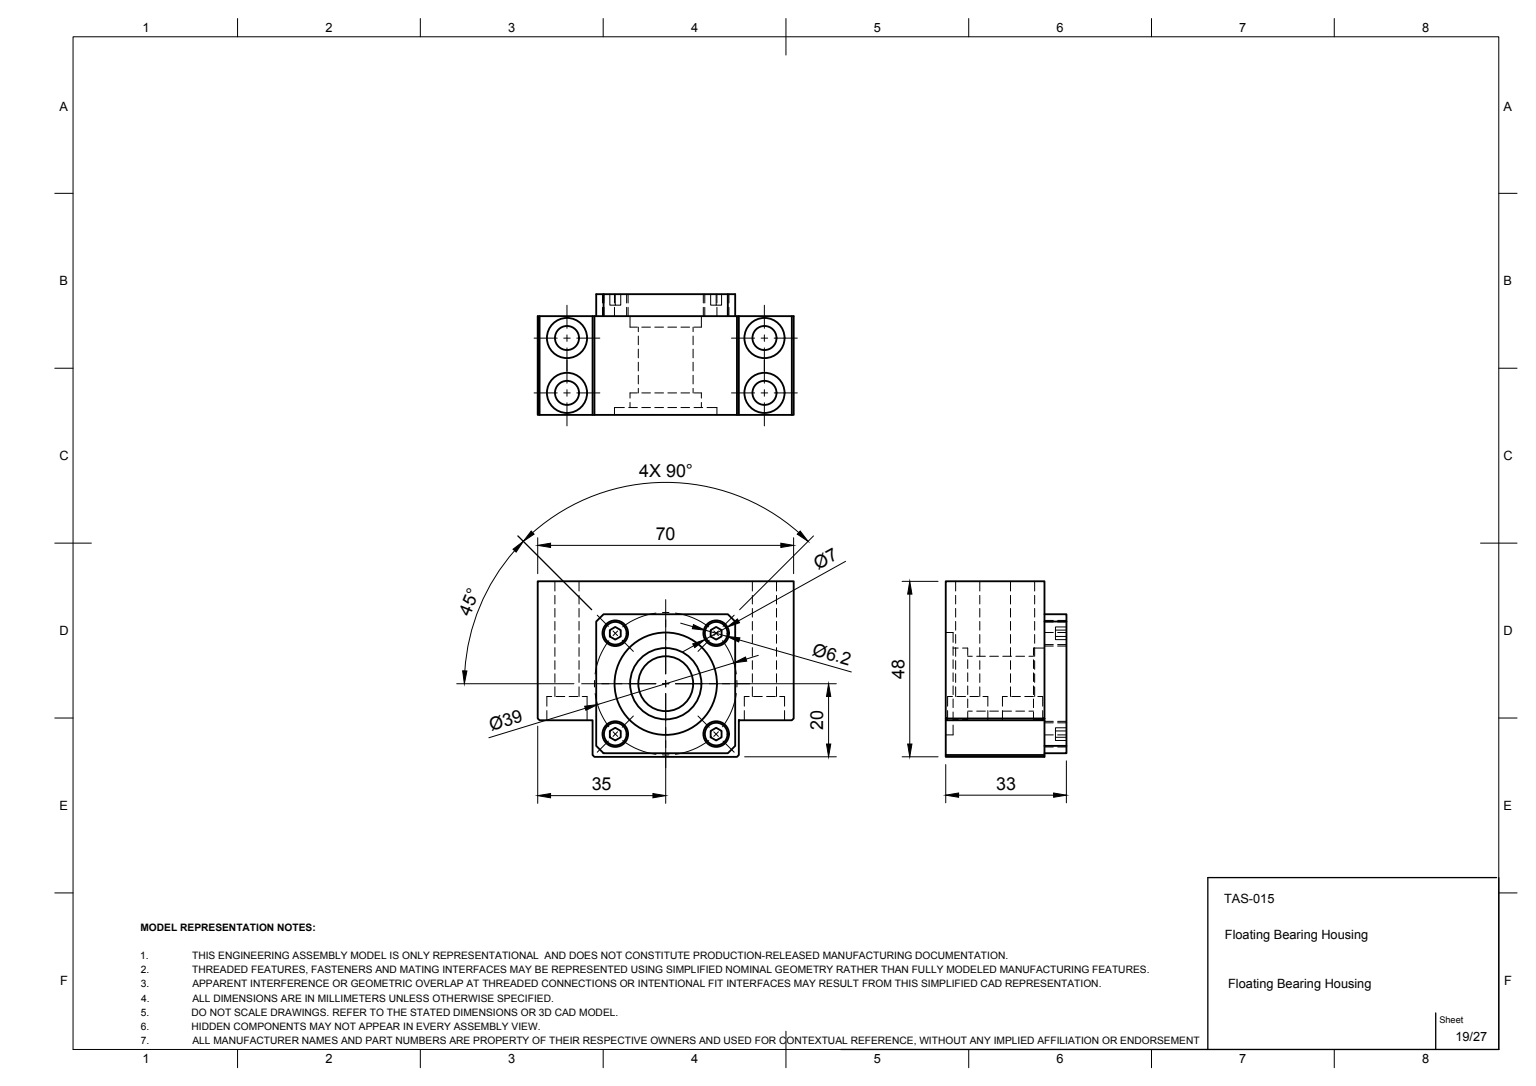
ISO-10303-21;
HEADER;
/* Generated by software containing ST-Developer
 * from STEP Tools, Inc. (www.steptools.com) 
 */

FILE_DESCRIPTION(
/* description */ ('STEP AP214'),
/* implementation_level */ '2;1');

FILE_NAME(
/* name */ 'Floating Bearing Housing.step',
/* time_stamp */ '2026-11-15T14:49:54-08:00',
/* author */ (''),
/* organization */ (''),
/* preprocessor_version */ 'ST-DEVELOPER v20.2',
/* originating_system */ 'Autodesk Translation Framework v15.17.0.0',
/* authorisation */ '');

FILE_SCHEMA (('AUTOMOTIVE_DESIGN { 1 0 10303 214 3 1 1 }'));
ENDSEC;

DATA;
#10=MECHANICAL_DESIGN_GEOMETRIC_PRESENTATION_REPRESENTATION('',(#1111),#66721);
#1049=SHAPE_REPRESENTATION_RELATIONSHIP('SRR','None',#66910,#1080);
#1080=ADVANCED_BREP_SHAPE_REPRESENTATION('',(#1146),#66701);
#1111=STYLED_ITEM('',(#67095),#1146);
#1146=MANIFOLD_SOLID_BREP('Body1',#25677);
#1342=FACE_BOUND('',#4614,.T.);
#1343=FACE_BOUND('',#4616,.T.);
#1344=FACE_BOUND('',#4618,.T.);
#1345=FACE_BOUND('',#4620,.T.);
#1346=FACE_BOUND('',#4622,.T.);
#1347=FACE_BOUND('',#4624,.T.);
#1348=FACE_BOUND('',#4625,.T.);
#1349=FACE_BOUND('',#4629,.T.);
#1350=FACE_BOUND('',#4630,.T.);
#1351=FACE_BOUND('',#4631,.T.);
#1352=FACE_BOUND('',#4632,.T.);
#1353=FACE_BOUND('',#4636,.T.);
#1354=FACE_BOUND('',#4637,.T.);
#1355=FACE_BOUND('',#4644,.T.);
#1356=FACE_BOUND('',#4646,.T.);
#1357=FACE_BOUND('',#4648,.T.);
#1358=FACE_BOUND('',#4650,.T.);
#1359=FACE_BOUND('',#4652,.T.);
#1360=FACE_BOUND('',#4654,.T.);
#1361=FACE_BOUND('',#4655,.T.);
#1362=FACE_BOUND('',#4656,.T.);
#1363=FACE_BOUND('',#4657,.T.);
#1364=FACE_BOUND('',#4658,.T.);
#1365=FACE_BOUND('',#4668,.T.);
#1366=FACE_BOUND('',#4670,.T.);
#1367=FACE_BOUND('',#4672,.T.);
#1368=FACE_BOUND('',#4674,.T.);
#1369=FACE_BOUND('',#4704,.T.);
#1370=FACE_BOUND('',#4706,.T.);
#1371=FACE_BOUND('',#4708,.T.);
#1372=FACE_BOUND('',#4710,.T.);
#1915=PLANE('',#27535);
#1916=PLANE('',#27536);
#1917=PLANE('',#27537);
#1918=PLANE('',#27538);
#1919=PLANE('',#27539);
#1920=PLANE('',#27540);
#1921=PLANE('',#27541);
#1922=PLANE('',#27542);
#1923=PLANE('',#27543);
#1924=PLANE('',#27544);
#1925=PLANE('',#27545);
#1926=PLANE('',#27546);
#1927=PLANE('',#27547);
#1928=PLANE('',#27548);
#1929=PLANE('',#27549);
#1930=PLANE('',#27550);
#1931=PLANE('',#27551);
#1932=PLANE('',#27552);
#1933=PLANE('',#27553);
#1934=PLANE('',#27554);
#1935=PLANE('',#27555);
#1936=PLANE('',#27556);
#1937=PLANE('',#27557);
#1938=PLANE('',#27558);
#1939=PLANE('',#27559);
#1940=PLANE('',#27560);
#1941=PLANE('',#27561);
#1942=PLANE('',#27562);
#1943=PLANE('',#27563);
#1944=PLANE('',#27564);
#1945=PLANE('',#27565);
#1946=PLANE('',#27566);
#1947=PLANE('',#27567);
#1948=PLANE('',#27568);
#1949=PLANE('',#27569);
#1950=PLANE('',#27570);
#1951=PLANE('',#27571);
#1952=PLANE('',#27572);
#1953=PLANE('',#27573);
#1954=PLANE('',#27574);
#1955=PLANE('',#27575);
#1956=PLANE('',#27576);
#1957=PLANE('',#27577);
#1958=PLANE('',#27578);
#1959=PLANE('',#27579);
#1960=PLANE('',#27580);
#1961=PLANE('',#27581);
#1962=PLANE('',#27582);
#1963=PLANE('',#27583);
#1964=PLANE('',#27584);
#1965=PLANE('',#27585);
#1966=PLANE('',#27586);
#1967=PLANE('',#27587);
#1968=PLANE('',#27588);
#1969=PLANE('',#27589);
#1970=PLANE('',#27590);
#1971=PLANE('',#27591);
#1972=PLANE('',#27592);
#1973=PLANE('',#27593);
#1974=PLANE('',#27594);
#1975=PLANE('',#27595);
#1976=PLANE('',#27596);
#1977=PLANE('',#27597);
#1978=PLANE('',#27598);
#1979=PLANE('',#27599);
#1980=PLANE('',#27600);
#1981=PLANE('',#27601);
#2976=FACE_OUTER_BOUND('',#4592,.T.);
#2977=FACE_OUTER_BOUND('',#4593,.T.);
#2978=FACE_OUTER_BOUND('',#4594,.T.);
#2979=FACE_OUTER_BOUND('',#4595,.T.);
#2980=FACE_OUTER_BOUND('',#4596,.T.);
#2981=FACE_OUTER_BOUND('',#4597,.T.);
#2982=FACE_OUTER_BOUND('',#4598,.T.);
#2983=FACE_OUTER_BOUND('',#4599,.T.);
#2984=FACE_OUTER_BOUND('',#4600,.T.);
#2985=FACE_OUTER_BOUND('',#4601,.T.);
#2986=FACE_OUTER_BOUND('',#4602,.T.);
#2987=FACE_OUTER_BOUND('',#4603,.T.);
#2988=FACE_OUTER_BOUND('',#4604,.T.);
#2989=FACE_OUTER_BOUND('',#4605,.T.);
#2990=FACE_OUTER_BOUND('',#4606,.T.);
#2991=FACE_OUTER_BOUND('',#4607,.T.);
#2992=FACE_OUTER_BOUND('',#4608,.T.);
#2993=FACE_OUTER_BOUND('',#4609,.T.);
#2994=FACE_OUTER_BOUND('',#4610,.T.);
#2995=FACE_OUTER_BOUND('',#4611,.T.);
#2996=FACE_OUTER_BOUND('',#4612,.T.);
#2997=FACE_OUTER_BOUND('',#4613,.T.);
#2998=FACE_OUTER_BOUND('',#4615,.T.);
#2999=FACE_OUTER_BOUND('',#4617,.T.);
#3000=FACE_OUTER_BOUND('',#4619,.T.);
#3001=FACE_OUTER_BOUND('',#4621,.T.);
#3002=FACE_OUTER_BOUND('',#4623,.T.);
#3003=FACE_OUTER_BOUND('',#4626,.T.);
#3004=FACE_OUTER_BOUND('',#4627,.T.);
#3005=FACE_OUTER_BOUND('',#4628,.T.);
#3006=FACE_OUTER_BOUND('',#4633,.T.);
#3007=FACE_OUTER_BOUND('',#4634,.T.);
#3008=FACE_OUTER_BOUND('',#4635,.T.);
#3009=FACE_OUTER_BOUND('',#4638,.T.);
#3010=FACE_OUTER_BOUND('',#4639,.T.);
#3011=FACE_OUTER_BOUND('',#4640,.T.);
#3012=FACE_OUTER_BOUND('',#4641,.T.);
#3013=FACE_OUTER_BOUND('',#4642,.T.);
#3014=FACE_OUTER_BOUND('',#4643,.T.);
#3015=FACE_OUTER_BOUND('',#4645,.T.);
#3016=FACE_OUTER_BOUND('',#4647,.T.);
#3017=FACE_OUTER_BOUND('',#4649,.T.);
#3018=FACE_OUTER_BOUND('',#4651,.T.);
#3019=FACE_OUTER_BOUND('',#4653,.T.);
#3020=FACE_OUTER_BOUND('',#4659,.T.);
#3021=FACE_OUTER_BOUND('',#4660,.T.);
#3022=FACE_OUTER_BOUND('',#4661,.T.);
#3023=FACE_OUTER_BOUND('',#4662,.T.);
#3024=FACE_OUTER_BOUND('',#4663,.T.);
#3025=FACE_OUTER_BOUND('',#4664,.T.);
#3026=FACE_OUTER_BOUND('',#4665,.T.);
#3027=FACE_OUTER_BOUND('',#4666,.T.);
#3028=FACE_OUTER_BOUND('',#4667,.T.);
#3029=FACE_OUTER_BOUND('',#4669,.T.);
#3030=FACE_OUTER_BOUND('',#4671,.T.);
#3031=FACE_OUTER_BOUND('',#4673,.T.);
#3032=FACE_OUTER_BOUND('',#4675,.T.);
#3033=FACE_OUTER_BOUND('',#4676,.T.);
#3034=FACE_OUTER_BOUND('',#4677,.T.);
#3035=FACE_OUTER_BOUND('',#4678,.T.);
#3036=FACE_OUTER_BOUND('',#4679,.T.);
#3037=FACE_OUTER_BOUND('',#4680,.T.);
#3038=FACE_OUTER_BOUND('',#4681,.T.);
#3039=FACE_OUTER_BOUND('',#4682,.T.);
#3040=FACE_OUTER_BOUND('',#4683,.T.);
#3041=FACE_OUTER_BOUND('',#4684,.T.);
#3042=FACE_OUTER_BOUND('',#4685,.T.);
#3043=FACE_OUTER_BOUND('',#4686,.T.);
#3044=FACE_OUTER_BOUND('',#4687,.T.);
#3045=FACE_OUTER_BOUND('',#4688,.T.);
#3046=FACE_OUTER_BOUND('',#4689,.T.);
#3047=FACE_OUTER_BOUND('',#4690,.T.);
#3048=FACE_OUTER_BOUND('',#4691,.T.);
#3049=FACE_OUTER_BOUND('',#4692,.T.);
#3050=FACE_OUTER_BOUND('',#4693,.T.);
#3051=FACE_OUTER_BOUND('',#4694,.T.);
#3052=FACE_OUTER_BOUND('',#4695,.T.);
#3053=FACE_OUTER_BOUND('',#4696,.T.);
#3054=FACE_OUTER_BOUND('',#4697,.T.);
#3055=FACE_OUTER_BOUND('',#4698,.T.);
#3056=FACE_OUTER_BOUND('',#4699,.T.);
#3057=FACE_OUTER_BOUND('',#4700,.T.);
#3058=FACE_OUTER_BOUND('',#4701,.T.);
#3059=FACE_OUTER_BOUND('',#4702,.T.);
#3060=FACE_OUTER_BOUND('',#4703,.T.);
#3061=FACE_OUTER_BOUND('',#4705,.T.);
#3062=FACE_OUTER_BOUND('',#4707,.T.);
#3063=FACE_OUTER_BOUND('',#4709,.T.);
#4592=EDGE_LOOP('',(#20414,#20415,#20416,#20417));
#4593=EDGE_LOOP('',(#20418,#20419,#20420,#20421));
#4594=EDGE_LOOP('',(#20422,#20423,#20424,#20425));
#4595=EDGE_LOOP('',(#20426,#20427,#20428,#20429));
#4596=EDGE_LOOP('',(#20430,#20431,#20432,#20433));
#4597=EDGE_LOOP('',(#20434,#20435,#20436,#20437));
#4598=EDGE_LOOP('',(#20438,#20439,#20440,#20441));
#4599=EDGE_LOOP('',(#20442,#20443,#20444,#20445));
#4600=EDGE_LOOP('',(#20446,#20447,#20448,#20449));
#4601=EDGE_LOOP('',(#20450,#20451,#20452,#20453));
#4602=EDGE_LOOP('',(#20454,#20455,#20456,#20457));
#4603=EDGE_LOOP('',(#20458,#20459,#20460,#20461));
#4604=EDGE_LOOP('',(#20462,#20463,#20464,#20465));
#4605=EDGE_LOOP('',(#20466,#20467,#20468,#20469));
#4606=EDGE_LOOP('',(#20470,#20471,#20472,#20473));
#4607=EDGE_LOOP('',(#20474,#20475,#20476,#20477));
#4608=EDGE_LOOP('',(#20478,#20479,#20480,#20481));
#4609=EDGE_LOOP('',(#20482,#20483,#20484,#20485));
#4610=EDGE_LOOP('',(#20486,#20487,#20488,#20489));
#4611=EDGE_LOOP('',(#20490,#20491,#20492,#20493));
#4612=EDGE_LOOP('',(#20494,#20495,#20496,#20497));
#4613=EDGE_LOOP('',(#20498));
#4614=EDGE_LOOP('',(#20499));
#4615=EDGE_LOOP('',(#20500));
#4616=EDGE_LOOP('',(#20501));
#4617=EDGE_LOOP('',(#20502));
#4618=EDGE_LOOP('',(#20503));
#4619=EDGE_LOOP('',(#20504));
#4620=EDGE_LOOP('',(#20505));
#4621=EDGE_LOOP('',(#20506,#20507,#20508,#20509,#20510,#20511,#20512,#20513,
#20514,#20515,#20516,#20517));
#4622=EDGE_LOOP('',(#20518,#20519,#20520,#20521,#20522,#20523,#20524,#20525));
#4623=EDGE_LOOP('',(#20526,#20527,#20528,#20529));
#4624=EDGE_LOOP('',(#20530));
#4625=EDGE_LOOP('',(#20531));
#4626=EDGE_LOOP('',(#20532,#20533,#20534,#20535));
#4627=EDGE_LOOP('',(#20536,#20537,#20538,#20539));
#4628=EDGE_LOOP('',(#20540,#20541,#20542,#20543));
#4629=EDGE_LOOP('',(#20544));
#4630=EDGE_LOOP('',(#20545));
#4631=EDGE_LOOP('',(#20546));
#4632=EDGE_LOOP('',(#20547));
#4633=EDGE_LOOP('',(#20548,#20549,#20550,#20551));
#4634=EDGE_LOOP('',(#20552,#20553,#20554,#20555));
#4635=EDGE_LOOP('',(#20556,#20557,#20558,#20559));
#4636=EDGE_LOOP('',(#20560));
#4637=EDGE_LOOP('',(#20561));
#4638=EDGE_LOOP('',(#20562,#20563,#20564,#20565));
#4639=EDGE_LOOP('',(#20566,#20567,#20568,#20569));
#4640=EDGE_LOOP('',(#20570,#20571,#20572,#20573));
#4641=EDGE_LOOP('',(#20574,#20575,#20576,#20577));
#4642=EDGE_LOOP('',(#20578,#20579,#20580,#20581));
#4643=EDGE_LOOP('',(#20582,#20583,#20584,#20585,#20586,#20587,#20588,#20589,
#20590,#20591,#20592,#20593));
#4644=EDGE_LOOP('',(#20594));
#4645=EDGE_LOOP('',(#20595));
#4646=EDGE_LOOP('',(#20596));
#4647=EDGE_LOOP('',(#20597));
#4648=EDGE_LOOP('',(#20598));
#4649=EDGE_LOOP('',(#20599));
#4650=EDGE_LOOP('',(#20600));
#4651=EDGE_LOOP('',(#20601));
#4652=EDGE_LOOP('',(#20602));
#4653=EDGE_LOOP('',(#20603,#20604,#20605,#20606,#20607,#20608,#20609,#20610));
#4654=EDGE_LOOP('',(#20611));
#4655=EDGE_LOOP('',(#20612));
#4656=EDGE_LOOP('',(#20613));
#4657=EDGE_LOOP('',(#20614));
#4658=EDGE_LOOP('',(#20615));
#4659=EDGE_LOOP('',(#20616,#20617,#20618,#20619));
#4660=EDGE_LOOP('',(#20620,#20621,#20622,#20623));
#4661=EDGE_LOOP('',(#20624,#20625,#20626,#20627));
#4662=EDGE_LOOP('',(#20628,#20629,#20630,#20631));
#4663=EDGE_LOOP('',(#20632,#20633,#20634,#20635));
#4664=EDGE_LOOP('',(#20636,#20637,#20638,#20639));
#4665=EDGE_LOOP('',(#20640,#20641,#20642,#20643));
#4666=EDGE_LOOP('',(#20644,#20645,#20646,#20647));
#4667=EDGE_LOOP('',(#20648));
#4668=EDGE_LOOP('',(#20649,#20650,#20651,#20652,#20653,#20654));
#4669=EDGE_LOOP('',(#20655));
#4670=EDGE_LOOP('',(#20656,#20657,#20658,#20659,#20660,#20661));
#4671=EDGE_LOOP('',(#20662));
#4672=EDGE_LOOP('',(#20663,#20664,#20665,#20666,#20667,#20668));
#4673=EDGE_LOOP('',(#20669));
#4674=EDGE_LOOP('',(#20670,#20671,#20672,#20673,#20674,#20675));
#4675=EDGE_LOOP('',(#20676,#20677,#20678,#20679));
#4676=EDGE_LOOP('',(#20680,#20681,#20682,#20683));
#4677=EDGE_LOOP('',(#20684,#20685,#20686,#20687));
#4678=EDGE_LOOP('',(#20688,#20689,#20690,#20691));
#4679=EDGE_LOOP('',(#20692,#20693,#20694,#20695));
#4680=EDGE_LOOP('',(#20696,#20697,#20698,#20699));
#4681=EDGE_LOOP('',(#20700,#20701,#20702,#20703,#20704,#20705));
#4682=EDGE_LOOP('',(#20706,#20707,#20708,#20709));
#4683=EDGE_LOOP('',(#20710,#20711,#20712,#20713));
#4684=EDGE_LOOP('',(#20714,#20715,#20716,#20717));
#4685=EDGE_LOOP('',(#20718,#20719,#20720,#20721));
#4686=EDGE_LOOP('',(#20722,#20723,#20724,#20725));
#4687=EDGE_LOOP('',(#20726,#20727,#20728,#20729));
#4688=EDGE_LOOP('',(#20730,#20731,#20732,#20733,#20734,#20735));
#4689=EDGE_LOOP('',(#20736,#20737,#20738,#20739));
#4690=EDGE_LOOP('',(#20740,#20741,#20742,#20743));
#4691=EDGE_LOOP('',(#20744,#20745,#20746,#20747));
#4692=EDGE_LOOP('',(#20748,#20749,#20750,#20751));
#4693=EDGE_LOOP('',(#20752,#20753,#20754,#20755));
#4694=EDGE_LOOP('',(#20756,#20757,#20758,#20759));
#4695=EDGE_LOOP('',(#20760,#20761,#20762,#20763,#20764,#20765));
#4696=EDGE_LOOP('',(#20766,#20767,#20768,#20769));
#4697=EDGE_LOOP('',(#20770,#20771,#20772,#20773));
#4698=EDGE_LOOP('',(#20774,#20775,#20776,#20777));
#4699=EDGE_LOOP('',(#20778,#20779,#20780,#20781));
#4700=EDGE_LOOP('',(#20782,#20783,#20784,#20785));
#4701=EDGE_LOOP('',(#20786,#20787,#20788,#20789));
#4702=EDGE_LOOP('',(#20790,#20791,#20792,#20793,#20794,#20795));
#4703=EDGE_LOOP('',(#20796));
#4704=EDGE_LOOP('',(#20797));
#4705=EDGE_LOOP('',(#20798));
#4706=EDGE_LOOP('',(#20799));
#4707=EDGE_LOOP('',(#20800));
#4708=EDGE_LOOP('',(#20801));
#4709=EDGE_LOOP('',(#20802));
#4710=EDGE_LOOP('',(#20803));
#6658=LINE('',#40429,#8647);
#6659=LINE('',#40435,#8648);
#6660=LINE('',#40441,#8649);
#6661=LINE('',#40447,#8650);
#6662=LINE('',#40453,#8651);
#6663=LINE('',#40459,#8652);
#6664=LINE('',#40465,#8653);
#6665=LINE('',#40471,#8654);
#6666=LINE('',#40477,#8655);
#6667=LINE('',#40483,#8656);
#6668=LINE('',#40489,#8657);
#6669=LINE('',#40495,#8658);
#6670=LINE('',#40501,#8659);
#6671=LINE('',#40507,#8660);
#6672=LINE('',#40513,#8661);
#6673=LINE('',#40519,#8662);
#6674=LINE('',#40525,#8663);
#6675=LINE('',#40531,#8664);
#6676=LINE('',#40537,#8665);
#6677=LINE('',#40543,#8666);
#6678=LINE('',#40549,#8667);
#6679=LINE('',#40558,#8668);
#6680=LINE('',#40560,#8669);
#6681=LINE('',#40562,#8670);
#6682=LINE('',#40564,#8671);
#6683=LINE('',#40566,#8672);
#6684=LINE('',#40568,#8673);
#6685=LINE('',#40570,#8674);
#6686=LINE('',#40572,#8675);
#6687=LINE('',#40574,#8676);
#6688=LINE('',#40576,#8677);
#6689=LINE('',#40578,#8678);
#6690=LINE('',#40579,#8679);
#6691=LINE('',#40582,#8680);
#6692=LINE('',#40584,#8681);
#6693=LINE('',#40586,#8682);
#6694=LINE('',#40588,#8683);
#6695=LINE('',#40590,#8684);
#6696=LINE('',#40592,#8685);
#6697=LINE('',#40594,#8686);
#6698=LINE('',#40595,#8687);
#6699=LINE('',#40599,#8688);
#6700=LINE('',#40600,#8689);
#6701=LINE('',#40601,#8690);
#6702=LINE('',#40604,#8691);
#6703=LINE('',#40605,#8692);
#6704=LINE('',#40608,#8693);
#6705=LINE('',#40609,#8694);
#6706=LINE('',#40612,#8695);
#6707=LINE('',#40613,#8696);
#6708=LINE('',#40616,#8697);
#6709=LINE('',#40617,#8698);
#6710=LINE('',#40620,#8699);
#6711=LINE('',#40621,#8700);
#6712=LINE('',#40624,#8701);
#6713=LINE('',#40625,#8702);
#6714=LINE('',#40628,#8703);
#6715=LINE('',#40629,#8704);
#6716=LINE('',#40632,#8705);
#6717=LINE('',#40633,#8706);
#6718=LINE('',#40636,#8707);
#6719=LINE('',#40637,#8708);
#6720=LINE('',#40640,#8709);
#6721=LINE('',#40641,#8710);
#6722=LINE('',#40643,#8711);
#6723=LINE('',#40652,#8712);
#6724=LINE('',#40654,#8713);
#6725=LINE('',#40656,#8714);
#6726=LINE('',#40658,#8715);
#6727=LINE('',#40660,#8716);
#6728=LINE('',#40662,#8717);
#6729=LINE('',#40664,#8718);
#6730=LINE('',#40665,#8719);
#6731=LINE('',#40667,#8720);
#6732=LINE('',#40668,#8721);
#6733=LINE('',#40670,#8722);
#6734=LINE('',#40672,#8723);
#6735=LINE('',#40674,#8724);
#6736=LINE('',#40676,#8725);
#6737=LINE('',#40678,#8726);
#6738=LINE('',#40680,#8727);
#6739=LINE('',#40685,#8728);
#6740=LINE('',#40687,#8729);
#6741=LINE('',#40689,#8730);
#6742=LINE('',#40691,#8731);
#6743=LINE('',#40693,#8732);
#6744=LINE('',#40694,#8733);
#6745=LINE('',#40698,#8734);
#6746=LINE('',#40700,#8735);
#6747=LINE('',#40702,#8736);
#6748=LINE('',#40704,#8737);
#6749=LINE('',#40706,#8738);
#6750=LINE('',#40707,#8739);
#6751=LINE('',#40711,#8740);
#6752=LINE('',#40713,#8741);
#6753=LINE('',#40715,#8742);
#6754=LINE('',#40717,#8743);
#6755=LINE('',#40719,#8744);
#6756=LINE('',#40720,#8745);
#6757=LINE('',#40724,#8746);
#6758=LINE('',#40726,#8747);
#6759=LINE('',#40728,#8748);
#6760=LINE('',#40730,#8749);
#6761=LINE('',#40732,#8750);
#6762=LINE('',#40733,#8751);
#6763=LINE('',#40736,#8752);
#6764=LINE('',#40738,#8753);
#6765=LINE('',#40739,#8754);
#6766=LINE('',#40742,#8755);
#6767=LINE('',#40743,#8756);
#6768=LINE('',#40746,#8757);
#6769=LINE('',#40747,#8758);
#6770=LINE('',#40750,#8759);
#6771=LINE('',#40751,#8760);
#6772=LINE('',#40754,#8761);
#6773=LINE('',#40755,#8762);
#6774=LINE('',#40757,#8763);
#6775=LINE('',#40761,#8764);
#6776=LINE('',#40763,#8765);
#6777=LINE('',#40764,#8766);
#6778=LINE('',#40767,#8767);
#6779=LINE('',#40768,#8768);
#6780=LINE('',#40771,#8769);
#6781=LINE('',#40772,#8770);
#6782=LINE('',#40775,#8771);
#6783=LINE('',#40776,#8772);
#6784=LINE('',#40779,#8773);
#6785=LINE('',#40780,#8774);
#6786=LINE('',#40782,#8775);
#6787=LINE('',#40786,#8776);
#6788=LINE('',#40788,#8777);
#6789=LINE('',#40789,#8778);
#6790=LINE('',#40792,#8779);
#6791=LINE('',#40793,#8780);
#6792=LINE('',#40796,#8781);
#6793=LINE('',#40797,#8782);
#6794=LINE('',#40800,#8783);
#6795=LINE('',#40801,#8784);
#6796=LINE('',#40804,#8785);
#6797=LINE('',#40805,#8786);
#6798=LINE('',#40807,#8787);
#6799=LINE('',#40811,#8788);
#6800=LINE('',#40813,#8789);
#6801=LINE('',#40814,#8790);
#6802=LINE('',#40817,#8791);
#6803=LINE('',#40818,#8792);
#6804=LINE('',#40821,#8793);
#6805=LINE('',#40822,#8794);
#6806=LINE('',#40825,#8795);
#6807=LINE('',#40826,#8796);
#6808=LINE('',#40829,#8797);
#6809=LINE('',#40830,#8798);
#6810=LINE('',#40832,#8799);
#8647=VECTOR('',#32797,14.);
#8648=VECTOR('',#32804,9.75);
#8649=VECTOR('',#32811,7.5);
#8650=VECTOR('',#32818,9.75);
#8651=VECTOR('',#32825,14.);
#8652=VECTOR('',#32832,3.1);
#8653=VECTOR('',#32839,3.1);
#8654=VECTOR('',#32846,3.1);
#8655=VECTOR('',#32853,3.1);
#8656=VECTOR('',#32860,3.50000000000001);
#8657=VECTOR('',#32867,3.5);
#8658=VECTOR('',#32874,3.50000000000001);
#8659=VECTOR('',#32881,3.50000000000001);
#8660=VECTOR('',#32888,5.5);
#8661=VECTOR('',#32895,3.3);
#8662=VECTOR('',#32902,5.5);
#8663=VECTOR('',#32909,3.3);
#8664=VECTOR('',#32916,5.5);
#8665=VECTOR('',#32923,3.3);
#8666=VECTOR('',#32930,5.5);
#8667=VECTOR('',#32937,3.3);
#8668=VECTOR('',#32950,1000.);
#8669=VECTOR('',#32951,1000.);
#8670=VECTOR('',#32952,1000.);
#8671=VECTOR('',#32953,1000.);
#8672=VECTOR('',#32954,1000.);
#8673=VECTOR('',#32955,1000.);
#8674=VECTOR('',#32956,1000.);
#8675=VECTOR('',#32957,1000.);
#8676=VECTOR('',#32958,1000.);
#8677=VECTOR('',#32959,1000.);
#8678=VECTOR('',#32960,1000.);
#8679=VECTOR('',#32961,1000.);
#8680=VECTOR('',#32962,1000.);
#8681=VECTOR('',#32963,1000.);
#8682=VECTOR('',#32964,1000.);
#8683=VECTOR('',#32965,1000.);
#8684=VECTOR('',#32966,1000.);
#8685=VECTOR('',#32967,1000.);
#8686=VECTOR('',#32968,1000.);
#8687=VECTOR('',#32969,1000.);
#8688=VECTOR('',#32972,1000.);
#8689=VECTOR('',#32973,1000.);
#8690=VECTOR('',#32974,1000.);
#8691=VECTOR('',#32977,1000.);
#8692=VECTOR('',#32978,1000.);
#8693=VECTOR('',#32981,1000.);
#8694=VECTOR('',#32982,1000.);
#8695=VECTOR('',#32985,1000.);
#8696=VECTOR('',#32986,1000.);
#8697=VECTOR('',#32989,1000.);
#8698=VECTOR('',#32990,1000.);
#8699=VECTOR('',#32993,1000.);
#8700=VECTOR('',#32994,1000.);
#8701=VECTOR('',#32997,1000.);
#8702=VECTOR('',#32998,1000.);
#8703=VECTOR('',#33001,1000.);
#8704=VECTOR('',#33002,1000.);
#8705=VECTOR('',#33005,1000.);
#8706=VECTOR('',#33006,1000.);
#8707=VECTOR('',#33009,1000.);
#8708=VECTOR('',#33010,1000.);
#8709=VECTOR('',#33013,1000.);
#8710=VECTOR('',#33014,1000.);
#8711=VECTOR('',#33017,1000.);
#8712=VECTOR('',#33030,1000.);
#8713=VECTOR('',#33031,1000.);
#8714=VECTOR('',#33032,1000.);
#8715=VECTOR('',#33033,1000.);
#8716=VECTOR('',#33034,1000.);
#8717=VECTOR('',#33035,1000.);
#8718=VECTOR('',#33036,1000.);
#8719=VECTOR('',#33037,1000.);
#8720=VECTOR('',#33040,1000.);
#8721=VECTOR('',#33041,1000.);
#8722=VECTOR('',#33044,1000.);
#8723=VECTOR('',#33047,1000.);
#8724=VECTOR('',#33050,1000.);
#8725=VECTOR('',#33053,1000.);
#8726=VECTOR('',#33056,1000.);
#8727=VECTOR('',#33059,1000.);
#8728=VECTOR('',#33064,1000.);
#8729=VECTOR('',#33065,1000.);
#8730=VECTOR('',#33066,1000.);
#8731=VECTOR('',#33067,1000.);
#8732=VECTOR('',#33068,1000.);
#8733=VECTOR('',#33069,1000.);
#8734=VECTOR('',#33072,1000.);
#8735=VECTOR('',#33073,1000.);
#8736=VECTOR('',#33074,1000.);
#8737=VECTOR('',#33075,1000.);
#8738=VECTOR('',#33076,1000.);
#8739=VECTOR('',#33077,1000.);
#8740=VECTOR('',#33080,1000.);
#8741=VECTOR('',#33081,1000.);
#8742=VECTOR('',#33082,1000.);
#8743=VECTOR('',#33083,1000.);
#8744=VECTOR('',#33084,1000.);
#8745=VECTOR('',#33085,1000.);
#8746=VECTOR('',#33088,1000.);
#8747=VECTOR('',#33089,1000.);
#8748=VECTOR('',#33090,1000.);
#8749=VECTOR('',#33091,1000.);
#8750=VECTOR('',#33092,1000.);
#8751=VECTOR('',#33093,1000.);
#8752=VECTOR('',#33096,1000.);
#8753=VECTOR('',#33097,1000.);
#8754=VECTOR('',#33098,1000.);
#8755=VECTOR('',#33101,1000.);
#8756=VECTOR('',#33102,1000.);
#8757=VECTOR('',#33105,1000.);
#8758=VECTOR('',#33106,1000.);
#8759=VECTOR('',#33109,1000.);
#8760=VECTOR('',#33110,1000.);
#8761=VECTOR('',#33113,1000.);
#8762=VECTOR('',#33114,1000.);
#8763=VECTOR('',#33117,1000.);
#8764=VECTOR('',#33122,1000.);
#8765=VECTOR('',#33123,1000.);
#8766=VECTOR('',#33124,1000.);
#8767=VECTOR('',#33127,1000.);
#8768=VECTOR('',#33128,1000.);
#8769=VECTOR('',#33131,1000.);
#8770=VECTOR('',#33132,1000.);
#8771=VECTOR('',#33135,1000.);
#8772=VECTOR('',#33136,1000.);
#8773=VECTOR('',#33139,1000.);
#8774=VECTOR('',#33140,1000.);
#8775=VECTOR('',#33143,1000.);
#8776=VECTOR('',#33148,1000.);
#8777=VECTOR('',#33149,1000.);
#8778=VECTOR('',#33150,1000.);
#8779=VECTOR('',#33153,1000.);
#8780=VECTOR('',#33154,1000.);
#8781=VECTOR('',#33157,1000.);
#8782=VECTOR('',#33158,1000.);
#8783=VECTOR('',#33161,1000.);
#8784=VECTOR('',#33162,1000.);
#8785=VECTOR('',#33165,1000.);
#8786=VECTOR('',#33166,1000.);
#8787=VECTOR('',#33169,1000.);
#8788=VECTOR('',#33174,1000.);
#8789=VECTOR('',#33175,1000.);
#8790=VECTOR('',#33176,1000.);
#8791=VECTOR('',#33179,1000.);
#8792=VECTOR('',#33180,1000.);
#8793=VECTOR('',#33183,1000.);
#8794=VECTOR('',#33184,1000.);
#8795=VECTOR('',#33187,1000.);
#8796=VECTOR('',#33188,1000.);
#8797=VECTOR('',#33191,1000.);
#8798=VECTOR('',#33192,1000.);
#8799=VECTOR('',#33195,1000.);
#10074=CIRCLE('',#27473,14.);
#10075=CIRCLE('',#27474,14.);
#10076=CIRCLE('',#27476,9.75);
#10077=CIRCLE('',#27477,9.75);
#10078=CIRCLE('',#27479,7.5);
#10079=CIRCLE('',#27480,7.5);
#10080=CIRCLE('',#27482,9.75);
#10081=CIRCLE('',#27483,9.75);
#10082=CIRCLE('',#27485,14.);
#10083=CIRCLE('',#27486,14.);
#10084=CIRCLE('',#27488,3.1);
#10085=CIRCLE('',#27489,3.1);
#10086=CIRCLE('',#27491,3.1);
#10087=CIRCLE('',#27492,3.1);
#10088=CIRCLE('',#27494,3.1);
#10089=CIRCLE('',#27495,3.1);
#10090=CIRCLE('',#27497,3.1);
#10091=CIRCLE('',#27498,3.1);
#10092=CIRCLE('',#27500,3.50000000000001);
#10093=CIRCLE('',#27501,3.50000000000001);
#10094=CIRCLE('',#27503,3.5);
#10095=CIRCLE('',#27504,3.5);
#10096=CIRCLE('',#27506,3.50000000000001);
#10097=CIRCLE('',#27507,3.50000000000001);
#10098=CIRCLE('',#27509,3.50000000000001);
#10099=CIRCLE('',#27510,3.50000000000001);
#10100=CIRCLE('',#27512,5.5);
#10101=CIRCLE('',#27513,5.5);
#10102=CIRCLE('',#27515,3.29999999999999);
#10103=CIRCLE('',#27516,3.3);
#10104=CIRCLE('',#27518,5.5);
#10105=CIRCLE('',#27519,5.5);
#10106=CIRCLE('',#27521,3.29999999999999);
#10107=CIRCLE('',#27522,3.3);
#10108=CIRCLE('',#27524,5.5);
#10109=CIRCLE('',#27525,5.5);
#10110=CIRCLE('',#27527,3.29999999999999);
#10111=CIRCLE('',#27528,3.3);
#10112=CIRCLE('',#27530,5.5);
#10113=CIRCLE('',#27531,5.5);
#10114=CIRCLE('',#27533,3.29999999999999);
#10115=CIRCLE('',#27534,3.3);
#11901=VERTEX_POINT('',#40426);
#11902=VERTEX_POINT('',#40428);
#11903=VERTEX_POINT('',#40432);
#11904=VERTEX_POINT('',#40434);
#11905=VERTEX_POINT('',#40438);
#11906=VERTEX_POINT('',#40440);
#11907=VERTEX_POINT('',#40444);
#11908=VERTEX_POINT('',#40446);
#11909=VERTEX_POINT('',#40450);
#11910=VERTEX_POINT('',#40452);
#11911=VERTEX_POINT('',#40456);
#11912=VERTEX_POINT('',#40458);
#11913=VERTEX_POINT('',#40462);
#11914=VERTEX_POINT('',#40464);
#11915=VERTEX_POINT('',#40468);
#11916=VERTEX_POINT('',#40470);
#11917=VERTEX_POINT('',#40474);
#11918=VERTEX_POINT('',#40476);
#11919=VERTEX_POINT('',#40480);
#11920=VERTEX_POINT('',#40482);
#11921=VERTEX_POINT('',#40486);
#11922=VERTEX_POINT('',#40488);
#11923=VERTEX_POINT('',#40492);
#11924=VERTEX_POINT('',#40494);
#11925=VERTEX_POINT('',#40498);
#11926=VERTEX_POINT('',#40500);
#11927=VERTEX_POINT('',#40504);
#11928=VERTEX_POINT('',#40506);
#11929=VERTEX_POINT('',#40510);
#11930=VERTEX_POINT('',#40512);
#11931=VERTEX_POINT('',#40516);
#11932=VERTEX_POINT('',#40518);
#11933=VERTEX_POINT('',#40522);
#11934=VERTEX_POINT('',#40524);
#11935=VERTEX_POINT('',#40528);
#11936=VERTEX_POINT('',#40530);
#11937=VERTEX_POINT('',#40534);
#11938=VERTEX_POINT('',#40536);
#11939=VERTEX_POINT('',#40540);
#11940=VERTEX_POINT('',#40542);
#11941=VERTEX_POINT('',#40546);
#11942=VERTEX_POINT('',#40548);
#11943=VERTEX_POINT('',#40556);
#11944=VERTEX_POINT('',#40557);
#11945=VERTEX_POINT('',#40559);
#11946=VERTEX_POINT('',#40561);
#11947=VERTEX_POINT('',#40563);
#11948=VERTEX_POINT('',#40565);
#11949=VERTEX_POINT('',#40567);
#11950=VERTEX_POINT('',#40569);
#11951=VERTEX_POINT('',#40571);
#11952=VERTEX_POINT('',#40573);
#11953=VERTEX_POINT('',#40575);
#11954=VERTEX_POINT('',#40577);
#11955=VERTEX_POINT('',#40580);
#11956=VERTEX_POINT('',#40581);
#11957=VERTEX_POINT('',#40583);
#11958=VERTEX_POINT('',#40585);
#11959=VERTEX_POINT('',#40587);
#11960=VERTEX_POINT('',#40589);
#11961=VERTEX_POINT('',#40591);
#11962=VERTEX_POINT('',#40593);
#11963=VERTEX_POINT('',#40597);
#11964=VERTEX_POINT('',#40598);
#11965=VERTEX_POINT('',#40603);
#11966=VERTEX_POINT('',#40607);
#11967=VERTEX_POINT('',#40611);
#11968=VERTEX_POINT('',#40615);
#11969=VERTEX_POINT('',#40619);
#11970=VERTEX_POINT('',#40623);
#11971=VERTEX_POINT('',#40627);
#11972=VERTEX_POINT('',#40631);
#11973=VERTEX_POINT('',#40635);
#11974=VERTEX_POINT('',#40639);
#11975=VERTEX_POINT('',#40650);
#11976=VERTEX_POINT('',#40651);
#11977=VERTEX_POINT('',#40653);
#11978=VERTEX_POINT('',#40655);
#11979=VERTEX_POINT('',#40657);
#11980=VERTEX_POINT('',#40659);
#11981=VERTEX_POINT('',#40661);
#11982=VERTEX_POINT('',#40663);
#11983=VERTEX_POINT('',#40683);
#11984=VERTEX_POINT('',#40684);
#11985=VERTEX_POINT('',#40686);
#11986=VERTEX_POINT('',#40688);
#11987=VERTEX_POINT('',#40690);
#11988=VERTEX_POINT('',#40692);
#11989=VERTEX_POINT('',#40696);
#11990=VERTEX_POINT('',#40697);
#11991=VERTEX_POINT('',#40699);
#11992=VERTEX_POINT('',#40701);
#11993=VERTEX_POINT('',#40703);
#11994=VERTEX_POINT('',#40705);
#11995=VERTEX_POINT('',#40709);
#11996=VERTEX_POINT('',#40710);
#11997=VERTEX_POINT('',#40712);
#11998=VERTEX_POINT('',#40714);
#11999=VERTEX_POINT('',#40716);
#12000=VERTEX_POINT('',#40718);
#12001=VERTEX_POINT('',#40722);
#12002=VERTEX_POINT('',#40723);
#12003=VERTEX_POINT('',#40725);
#12004=VERTEX_POINT('',#40727);
#12005=VERTEX_POINT('',#40729);
#12006=VERTEX_POINT('',#40731);
#12007=VERTEX_POINT('',#40735);
#12008=VERTEX_POINT('',#40737);
#12009=VERTEX_POINT('',#40741);
#12010=VERTEX_POINT('',#40745);
#12011=VERTEX_POINT('',#40749);
#12012=VERTEX_POINT('',#40753);
#12013=VERTEX_POINT('',#40760);
#12014=VERTEX_POINT('',#40762);
#12015=VERTEX_POINT('',#40766);
#12016=VERTEX_POINT('',#40770);
#12017=VERTEX_POINT('',#40774);
#12018=VERTEX_POINT('',#40778);
#12019=VERTEX_POINT('',#40785);
#12020=VERTEX_POINT('',#40787);
#12021=VERTEX_POINT('',#40791);
#12022=VERTEX_POINT('',#40795);
#12023=VERTEX_POINT('',#40799);
#12024=VERTEX_POINT('',#40803);
#12025=VERTEX_POINT('',#40810);
#12026=VERTEX_POINT('',#40812);
#12027=VERTEX_POINT('',#40816);
#12028=VERTEX_POINT('',#40820);
#12029=VERTEX_POINT('',#40824);
#12030=VERTEX_POINT('',#40828);
#14900=EDGE_CURVE('',#11901,#11901,#10074,.T.);
#14901=EDGE_CURVE('',#11901,#11902,#6658,.T.);
#14902=EDGE_CURVE('',#11902,#11902,#10075,.T.);
#14903=EDGE_CURVE('',#11903,#11903,#10076,.T.);
#14904=EDGE_CURVE('',#11903,#11904,#6659,.T.);
#14905=EDGE_CURVE('',#11904,#11904,#10077,.T.);
#14906=EDGE_CURVE('',#11905,#11905,#10078,.T.);
#14907=EDGE_CURVE('',#11905,#11906,#6660,.T.);
#14908=EDGE_CURVE('',#11906,#11906,#10079,.T.);
#14909=EDGE_CURVE('',#11907,#11907,#10080,.T.);
#14910=EDGE_CURVE('',#11907,#11908,#6661,.T.);
#14911=EDGE_CURVE('',#11908,#11908,#10081,.T.);
#14912=EDGE_CURVE('',#11909,#11909,#10082,.T.);
#14913=EDGE_CURVE('',#11909,#11910,#6662,.T.);
#14914=EDGE_CURVE('',#11910,#11910,#10083,.T.);
#14915=EDGE_CURVE('',#11911,#11911,#10084,.T.);
#14916=EDGE_CURVE('',#11911,#11912,#6663,.T.);
#14917=EDGE_CURVE('',#11912,#11912,#10085,.T.);
#14918=EDGE_CURVE('',#11913,#11913,#10086,.T.);
#14919=EDGE_CURVE('',#11913,#11914,#6664,.T.);
#14920=EDGE_CURVE('',#11914,#11914,#10087,.T.);
#14921=EDGE_CURVE('',#11915,#11915,#10088,.T.);
#14922=EDGE_CURVE('',#11915,#11916,#6665,.T.);
#14923=EDGE_CURVE('',#11916,#11916,#10089,.T.);
#14924=EDGE_CURVE('',#11917,#11917,#10090,.T.);
#14925=EDGE_CURVE('',#11917,#11918,#6666,.T.);
#14926=EDGE_CURVE('',#11918,#11918,#10091,.T.);
#14927=EDGE_CURVE('',#11919,#11919,#10092,.T.);
#14928=EDGE_CURVE('',#11919,#11920,#6667,.T.);
#14929=EDGE_CURVE('',#11920,#11920,#10093,.T.);
#14930=EDGE_CURVE('',#11921,#11921,#10094,.T.);
#14931=EDGE_CURVE('',#11921,#11922,#6668,.T.);
#14932=EDGE_CURVE('',#11922,#11922,#10095,.T.);
#14933=EDGE_CURVE('',#11923,#11923,#10096,.T.);
#14934=EDGE_CURVE('',#11923,#11924,#6669,.T.);
#14935=EDGE_CURVE('',#11924,#11924,#10097,.T.);
#14936=EDGE_CURVE('',#11925,#11925,#10098,.T.);
#14937=EDGE_CURVE('',#11925,#11926,#6670,.T.);
#14938=EDGE_CURVE('',#11926,#11926,#10099,.T.);
#14939=EDGE_CURVE('',#11927,#11927,#10100,.T.);
#14940=EDGE_CURVE('',#11927,#11928,#6671,.T.);
#14941=EDGE_CURVE('',#11928,#11928,#10101,.T.);
#14942=EDGE_CURVE('',#11929,#11929,#10102,.T.);
#14943=EDGE_CURVE('',#11929,#11930,#6672,.T.);
#14944=EDGE_CURVE('',#11930,#11930,#10103,.T.);
#14945=EDGE_CURVE('',#11931,#11931,#10104,.T.);
#14946=EDGE_CURVE('',#11931,#11932,#6673,.T.);
#14947=EDGE_CURVE('',#11932,#11932,#10105,.T.);
#14948=EDGE_CURVE('',#11933,#11933,#10106,.T.);
#14949=EDGE_CURVE('',#11933,#11934,#6674,.T.);
#14950=EDGE_CURVE('',#11934,#11934,#10107,.T.);
#14951=EDGE_CURVE('',#11935,#11935,#10108,.T.);
#14952=EDGE_CURVE('',#11935,#11936,#6675,.T.);
#14953=EDGE_CURVE('',#11936,#11936,#10109,.T.);
#14954=EDGE_CURVE('',#11937,#11937,#10110,.T.);
#14955=EDGE_CURVE('',#11937,#11938,#6676,.T.);
#14956=EDGE_CURVE('',#11938,#11938,#10111,.T.);
#14957=EDGE_CURVE('',#11939,#11939,#10112,.T.);
#14958=EDGE_CURVE('',#11939,#11940,#6677,.T.);
#14959=EDGE_CURVE('',#11940,#11940,#10113,.T.);
#14960=EDGE_CURVE('',#11941,#11941,#10114,.T.);
#14961=EDGE_CURVE('',#11941,#11942,#6678,.T.);
#14962=EDGE_CURVE('',#11942,#11942,#10115,.T.);
#14963=EDGE_CURVE('',#11943,#11944,#6679,.T.);
#14964=EDGE_CURVE('',#11944,#11945,#6680,.T.);
#14965=EDGE_CURVE('',#11945,#11946,#6681,.T.);
#14966=EDGE_CURVE('',#11946,#11947,#6682,.T.);
#14967=EDGE_CURVE('',#11947,#11948,#6683,.T.);
#14968=EDGE_CURVE('',#11948,#11949,#6684,.T.);
#14969=EDGE_CURVE('',#11949,#11950,#6685,.T.);
#14970=EDGE_CURVE('',#11950,#11951,#6686,.T.);
#14971=EDGE_CURVE('',#11951,#11952,#6687,.T.);
#14972=EDGE_CURVE('',#11952,#11953,#6688,.T.);
#14973=EDGE_CURVE('',#11953,#11954,#6689,.T.);
#14974=EDGE_CURVE('',#11954,#11943,#6690,.T.);
#14975=EDGE_CURVE('',#11955,#11956,#6691,.T.);
#14976=EDGE_CURVE('',#11957,#11955,#6692,.T.);
#14977=EDGE_CURVE('',#11958,#11957,#6693,.T.);
#14978=EDGE_CURVE('',#11959,#11958,#6694,.T.);
#14979=EDGE_CURVE('',#11960,#11959,#6695,.T.);
#14980=EDGE_CURVE('',#11961,#11960,#6696,.T.);
#14981=EDGE_CURVE('',#11962,#11961,#6697,.T.);
#14982=EDGE_CURVE('',#11956,#11962,#6698,.T.);
#14983=EDGE_CURVE('',#11963,#11964,#6699,.T.);
#14984=EDGE_CURVE('',#11944,#11964,#6700,.T.);
#14985=EDGE_CURVE('',#11943,#11963,#6701,.T.);
#14986=EDGE_CURVE('',#11964,#11965,#6702,.T.);
#14987=EDGE_CURVE('',#11945,#11965,#6703,.T.);
#14988=EDGE_CURVE('',#11965,#11966,#6704,.T.);
#14989=EDGE_CURVE('',#11946,#11966,#6705,.T.);
#14990=EDGE_CURVE('',#11966,#11967,#6706,.T.);
#14991=EDGE_CURVE('',#11947,#11967,#6707,.T.);
#14992=EDGE_CURVE('',#11967,#11968,#6708,.T.);
#14993=EDGE_CURVE('',#11948,#11968,#6709,.T.);
#14994=EDGE_CURVE('',#11968,#11969,#6710,.T.);
#14995=EDGE_CURVE('',#11949,#11969,#6711,.T.);
#14996=EDGE_CURVE('',#11969,#11970,#6712,.T.);
#14997=EDGE_CURVE('',#11950,#11970,#6713,.T.);
#14998=EDGE_CURVE('',#11970,#11971,#6714,.T.);
#14999=EDGE_CURVE('',#11951,#11971,#6715,.T.);
#15000=EDGE_CURVE('',#11971,#11972,#6716,.T.);
#15001=EDGE_CURVE('',#11952,#11972,#6717,.T.);
#15002=EDGE_CURVE('',#11972,#11973,#6718,.T.);
#15003=EDGE_CURVE('',#11953,#11973,#6719,.T.);
#15004=EDGE_CURVE('',#11973,#11974,#6720,.T.);
#15005=EDGE_CURVE('',#11954,#11974,#6721,.T.);
#15006=EDGE_CURVE('',#11974,#11963,#6722,.T.);
#15007=EDGE_CURVE('',#11975,#11976,#6723,.T.);
#15008=EDGE_CURVE('',#11976,#11977,#6724,.T.);
#15009=EDGE_CURVE('',#11977,#11978,#6725,.T.);
#15010=EDGE_CURVE('',#11978,#11979,#6726,.T.);
#15011=EDGE_CURVE('',#11979,#11980,#6727,.T.);
#15012=EDGE_CURVE('',#11980,#11981,#6728,.T.);
#15013=EDGE_CURVE('',#11981,#11982,#6729,.T.);
#15014=EDGE_CURVE('',#11982,#11975,#6730,.T.);
#15015=EDGE_CURVE('',#11976,#11955,#6731,.T.);
#15016=EDGE_CURVE('',#11975,#11957,#6732,.T.);
#15017=EDGE_CURVE('',#11977,#11956,#6733,.T.);
#15018=EDGE_CURVE('',#11978,#11962,#6734,.T.);
#15019=EDGE_CURVE('',#11979,#11961,#6735,.T.);
#15020=EDGE_CURVE('',#11980,#11960,#6736,.T.);
#15021=EDGE_CURVE('',#11981,#11959,#6737,.T.);
#15022=EDGE_CURVE('',#11982,#11958,#6738,.T.);
#15023=EDGE_CURVE('',#11983,#11984,#6739,.T.);
#15024=EDGE_CURVE('',#11985,#11983,#6740,.T.);
#15025=EDGE_CURVE('',#11986,#11985,#6741,.T.);
#15026=EDGE_CURVE('',#11987,#11986,#6742,.T.);
#15027=EDGE_CURVE('',#11988,#11987,#6743,.T.);
#15028=EDGE_CURVE('',#11984,#11988,#6744,.T.);
#15029=EDGE_CURVE('',#11989,#11990,#6745,.T.);
#15030=EDGE_CURVE('',#11991,#11989,#6746,.T.);
#15031=EDGE_CURVE('',#11992,#11991,#6747,.T.);
#15032=EDGE_CURVE('',#11993,#11992,#6748,.T.);
#15033=EDGE_CURVE('',#11994,#11993,#6749,.T.);
#15034=EDGE_CURVE('',#11990,#11994,#6750,.T.);
#15035=EDGE_CURVE('',#11995,#11996,#6751,.T.);
#15036=EDGE_CURVE('',#11997,#11995,#6752,.T.);
#15037=EDGE_CURVE('',#11998,#11997,#6753,.T.);
#15038=EDGE_CURVE('',#11999,#11998,#6754,.T.);
#15039=EDGE_CURVE('',#12000,#11999,#6755,.T.);
#15040=EDGE_CURVE('',#11996,#12000,#6756,.T.);
#15041=EDGE_CURVE('',#12001,#12002,#6757,.T.);
#15042=EDGE_CURVE('',#12003,#12001,#6758,.T.);
#15043=EDGE_CURVE('',#12004,#12003,#6759,.T.);
#15044=EDGE_CURVE('',#12005,#12004,#6760,.T.);
#15045=EDGE_CURVE('',#12006,#12005,#6761,.T.);
#15046=EDGE_CURVE('',#12002,#12006,#6762,.T.);
#15047=EDGE_CURVE('',#12007,#11984,#6763,.T.);
#15048=EDGE_CURVE('',#12008,#12007,#6764,.T.);
#15049=EDGE_CURVE('',#12008,#11983,#6765,.T.);
#15050=EDGE_CURVE('',#12009,#12008,#6766,.T.);
#15051=EDGE_CURVE('',#12009,#11985,#6767,.T.);
#15052=EDGE_CURVE('',#12010,#12009,#6768,.T.);
#15053=EDGE_CURVE('',#12010,#11986,#6769,.T.);
#15054=EDGE_CURVE('',#12011,#12010,#6770,.T.);
#15055=EDGE_CURVE('',#12011,#11987,#6771,.T.);
#15056=EDGE_CURVE('',#12012,#12011,#6772,.T.);
#15057=EDGE_CURVE('',#12012,#11988,#6773,.T.);
#15058=EDGE_CURVE('',#12007,#12012,#6774,.T.);
#15059=EDGE_CURVE('',#12013,#11990,#6775,.T.);
#15060=EDGE_CURVE('',#12014,#12013,#6776,.T.);
#15061=EDGE_CURVE('',#12014,#11989,#6777,.T.);
#15062=EDGE_CURVE('',#12015,#12014,#6778,.T.);
#15063=EDGE_CURVE('',#12015,#11991,#6779,.T.);
#15064=EDGE_CURVE('',#12016,#12015,#6780,.T.);
#15065=EDGE_CURVE('',#12016,#11992,#6781,.T.);
#15066=EDGE_CURVE('',#12017,#12016,#6782,.T.);
#15067=EDGE_CURVE('',#12017,#11993,#6783,.T.);
#15068=EDGE_CURVE('',#12018,#12017,#6784,.T.);
#15069=EDGE_CURVE('',#12018,#11994,#6785,.T.);
#15070=EDGE_CURVE('',#12013,#12018,#6786,.T.);
#15071=EDGE_CURVE('',#12019,#12002,#6787,.T.);
#15072=EDGE_CURVE('',#12020,#12019,#6788,.T.);
#15073=EDGE_CURVE('',#12020,#12001,#6789,.T.);
#15074=EDGE_CURVE('',#12021,#12020,#6790,.T.);
#15075=EDGE_CURVE('',#12021,#12003,#6791,.T.);
#15076=EDGE_CURVE('',#12022,#12021,#6792,.T.);
#15077=EDGE_CURVE('',#12022,#12004,#6793,.T.);
#15078=EDGE_CURVE('',#12023,#12022,#6794,.T.);
#15079=EDGE_CURVE('',#12023,#12005,#6795,.T.);
#15080=EDGE_CURVE('',#12024,#12023,#6796,.T.);
#15081=EDGE_CURVE('',#12024,#12006,#6797,.T.);
#15082=EDGE_CURVE('',#12019,#12024,#6798,.T.);
#15083=EDGE_CURVE('',#12025,#11996,#6799,.T.);
#15084=EDGE_CURVE('',#12026,#12025,#6800,.T.);
#15085=EDGE_CURVE('',#12026,#11995,#6801,.T.);
#15086=EDGE_CURVE('',#12027,#12026,#6802,.T.);
#15087=EDGE_CURVE('',#12027,#11997,#6803,.T.);
#15088=EDGE_CURVE('',#12028,#12027,#6804,.T.);
#15089=EDGE_CURVE('',#12028,#11998,#6805,.T.);
#15090=EDGE_CURVE('',#12029,#12028,#6806,.T.);
#15091=EDGE_CURVE('',#12029,#11999,#6807,.T.);
#15092=EDGE_CURVE('',#12030,#12029,#6808,.T.);
#15093=EDGE_CURVE('',#12030,#12000,#6809,.T.);
#15094=EDGE_CURVE('',#12025,#12030,#6810,.T.);
#20414=ORIENTED_EDGE('',*,*,#14900,.F.);
#20415=ORIENTED_EDGE('',*,*,#14901,.T.);
#20416=ORIENTED_EDGE('',*,*,#14902,.T.);
#20417=ORIENTED_EDGE('',*,*,#14901,.F.);
#20418=ORIENTED_EDGE('',*,*,#14903,.F.);
#20419=ORIENTED_EDGE('',*,*,#14904,.T.);
#20420=ORIENTED_EDGE('',*,*,#14905,.T.);
#20421=ORIENTED_EDGE('',*,*,#14904,.F.);
#20422=ORIENTED_EDGE('',*,*,#14906,.F.);
#20423=ORIENTED_EDGE('',*,*,#14907,.T.);
#20424=ORIENTED_EDGE('',*,*,#14908,.T.);
#20425=ORIENTED_EDGE('',*,*,#14907,.F.);
#20426=ORIENTED_EDGE('',*,*,#14909,.F.);
#20427=ORIENTED_EDGE('',*,*,#14910,.T.);
#20428=ORIENTED_EDGE('',*,*,#14911,.T.);
#20429=ORIENTED_EDGE('',*,*,#14910,.F.);
#20430=ORIENTED_EDGE('',*,*,#14912,.F.);
#20431=ORIENTED_EDGE('',*,*,#14913,.T.);
#20432=ORIENTED_EDGE('',*,*,#14914,.T.);
#20433=ORIENTED_EDGE('',*,*,#14913,.F.);
#20434=ORIENTED_EDGE('',*,*,#14915,.T.);
#20435=ORIENTED_EDGE('',*,*,#14916,.T.);
#20436=ORIENTED_EDGE('',*,*,#14917,.F.);
#20437=ORIENTED_EDGE('',*,*,#14916,.F.);
#20438=ORIENTED_EDGE('',*,*,#14918,.T.);
#20439=ORIENTED_EDGE('',*,*,#14919,.T.);
#20440=ORIENTED_EDGE('',*,*,#14920,.F.);
#20441=ORIENTED_EDGE('',*,*,#14919,.F.);
#20442=ORIENTED_EDGE('',*,*,#14921,.T.);
#20443=ORIENTED_EDGE('',*,*,#14922,.T.);
#20444=ORIENTED_EDGE('',*,*,#14923,.F.);
#20445=ORIENTED_EDGE('',*,*,#14922,.F.);
#20446=ORIENTED_EDGE('',*,*,#14924,.T.);
#20447=ORIENTED_EDGE('',*,*,#14925,.T.);
#20448=ORIENTED_EDGE('',*,*,#14926,.F.);
#20449=ORIENTED_EDGE('',*,*,#14925,.F.);
#20450=ORIENTED_EDGE('',*,*,#14927,.T.);
#20451=ORIENTED_EDGE('',*,*,#14928,.T.);
#20452=ORIENTED_EDGE('',*,*,#14929,.T.);
#20453=ORIENTED_EDGE('',*,*,#14928,.F.);
#20454=ORIENTED_EDGE('',*,*,#14930,.T.);
#20455=ORIENTED_EDGE('',*,*,#14931,.T.);
#20456=ORIENTED_EDGE('',*,*,#14932,.T.);
#20457=ORIENTED_EDGE('',*,*,#14931,.F.);
#20458=ORIENTED_EDGE('',*,*,#14933,.T.);
#20459=ORIENTED_EDGE('',*,*,#14934,.T.);
#20460=ORIENTED_EDGE('',*,*,#14935,.T.);
#20461=ORIENTED_EDGE('',*,*,#14934,.F.);
#20462=ORIENTED_EDGE('',*,*,#14936,.T.);
#20463=ORIENTED_EDGE('',*,*,#14937,.T.);
#20464=ORIENTED_EDGE('',*,*,#14938,.T.);
#20465=ORIENTED_EDGE('',*,*,#14937,.F.);
#20466=ORIENTED_EDGE('',*,*,#14939,.F.);
#20467=ORIENTED_EDGE('',*,*,#14940,.T.);
#20468=ORIENTED_EDGE('',*,*,#14941,.T.);
#20469=ORIENTED_EDGE('',*,*,#14940,.F.);
#20470=ORIENTED_EDGE('',*,*,#14942,.F.);
#20471=ORIENTED_EDGE('',*,*,#14943,.T.);
#20472=ORIENTED_EDGE('',*,*,#14944,.T.);
#20473=ORIENTED_EDGE('',*,*,#14943,.F.);
#20474=ORIENTED_EDGE('',*,*,#14945,.F.);
#20475=ORIENTED_EDGE('',*,*,#14946,.T.);
#20476=ORIENTED_EDGE('',*,*,#14947,.T.);
#20477=ORIENTED_EDGE('',*,*,#14946,.F.);
#20478=ORIENTED_EDGE('',*,*,#14948,.F.);
#20479=ORIENTED_EDGE('',*,*,#14949,.T.);
#20480=ORIENTED_EDGE('',*,*,#14950,.T.);
#20481=ORIENTED_EDGE('',*,*,#14949,.F.);
#20482=ORIENTED_EDGE('',*,*,#14951,.F.);
#20483=ORIENTED_EDGE('',*,*,#14952,.T.);
#20484=ORIENTED_EDGE('',*,*,#14953,.T.);
#20485=ORIENTED_EDGE('',*,*,#14952,.F.);
#20486=ORIENTED_EDGE('',*,*,#14954,.F.);
#20487=ORIENTED_EDGE('',*,*,#14955,.T.);
#20488=ORIENTED_EDGE('',*,*,#14956,.T.);
#20489=ORIENTED_EDGE('',*,*,#14955,.F.);
#20490=ORIENTED_EDGE('',*,*,#14957,.F.);
#20491=ORIENTED_EDGE('',*,*,#14958,.T.);
#20492=ORIENTED_EDGE('',*,*,#14959,.T.);
#20493=ORIENTED_EDGE('',*,*,#14958,.F.);
#20494=ORIENTED_EDGE('',*,*,#14960,.F.);
#20495=ORIENTED_EDGE('',*,*,#14961,.T.);
#20496=ORIENTED_EDGE('',*,*,#14962,.T.);
#20497=ORIENTED_EDGE('',*,*,#14961,.F.);
#20498=ORIENTED_EDGE('',*,*,#14932,.F.);
#20499=ORIENTED_EDGE('',*,*,#14915,.F.);
#20500=ORIENTED_EDGE('',*,*,#14929,.F.);
#20501=ORIENTED_EDGE('',*,*,#14918,.F.);
#20502=ORIENTED_EDGE('',*,*,#14935,.F.);
#20503=ORIENTED_EDGE('',*,*,#14921,.F.);
#20504=ORIENTED_EDGE('',*,*,#14938,.F.);
#20505=ORIENTED_EDGE('',*,*,#14924,.F.);
#20506=ORIENTED_EDGE('',*,*,#14963,.T.);
#20507=ORIENTED_EDGE('',*,*,#14964,.T.);
#20508=ORIENTED_EDGE('',*,*,#14965,.T.);
#20509=ORIENTED_EDGE('',*,*,#14966,.T.);
#20510=ORIENTED_EDGE('',*,*,#14967,.T.);
#20511=ORIENTED_EDGE('',*,*,#14968,.T.);
#20512=ORIENTED_EDGE('',*,*,#14969,.T.);
#20513=ORIENTED_EDGE('',*,*,#14970,.T.);
#20514=ORIENTED_EDGE('',*,*,#14971,.T.);
#20515=ORIENTED_EDGE('',*,*,#14972,.T.);
#20516=ORIENTED_EDGE('',*,*,#14973,.T.);
#20517=ORIENTED_EDGE('',*,*,#14974,.T.);
#20518=ORIENTED_EDGE('',*,*,#14975,.F.);
#20519=ORIENTED_EDGE('',*,*,#14976,.F.);
#20520=ORIENTED_EDGE('',*,*,#14977,.F.);
#20521=ORIENTED_EDGE('',*,*,#14978,.F.);
#20522=ORIENTED_EDGE('',*,*,#14979,.F.);
#20523=ORIENTED_EDGE('',*,*,#14980,.F.);
#20524=ORIENTED_EDGE('',*,*,#14981,.F.);
#20525=ORIENTED_EDGE('',*,*,#14982,.F.);
#20526=ORIENTED_EDGE('',*,*,#14983,.T.);
#20527=ORIENTED_EDGE('',*,*,#14984,.F.);
#20528=ORIENTED_EDGE('',*,*,#14963,.F.);
#20529=ORIENTED_EDGE('',*,*,#14985,.T.);
#20530=ORIENTED_EDGE('',*,*,#14947,.F.);
#20531=ORIENTED_EDGE('',*,*,#14959,.F.);
#20532=ORIENTED_EDGE('',*,*,#14986,.T.);
#20533=ORIENTED_EDGE('',*,*,#14987,.F.);
#20534=ORIENTED_EDGE('',*,*,#14964,.F.);
#20535=ORIENTED_EDGE('',*,*,#14984,.T.);
#20536=ORIENTED_EDGE('',*,*,#14988,.T.);
#20537=ORIENTED_EDGE('',*,*,#14989,.F.);
#20538=ORIENTED_EDGE('',*,*,#14965,.F.);
#20539=ORIENTED_EDGE('',*,*,#14987,.T.);
#20540=ORIENTED_EDGE('',*,*,#14990,.T.);
#20541=ORIENTED_EDGE('',*,*,#14991,.F.);
#20542=ORIENTED_EDGE('',*,*,#14966,.F.);
#20543=ORIENTED_EDGE('',*,*,#14989,.T.);
#20544=ORIENTED_EDGE('',*,*,#14942,.T.);
#20545=ORIENTED_EDGE('',*,*,#14948,.T.);
#20546=ORIENTED_EDGE('',*,*,#14954,.T.);
#20547=ORIENTED_EDGE('',*,*,#14960,.T.);
#20548=ORIENTED_EDGE('',*,*,#14992,.T.);
#20549=ORIENTED_EDGE('',*,*,#14993,.F.);
#20550=ORIENTED_EDGE('',*,*,#14967,.F.);
#20551=ORIENTED_EDGE('',*,*,#14991,.T.);
#20552=ORIENTED_EDGE('',*,*,#14994,.T.);
#20553=ORIENTED_EDGE('',*,*,#14995,.F.);
#20554=ORIENTED_EDGE('',*,*,#14968,.F.);
#20555=ORIENTED_EDGE('',*,*,#14993,.T.);
#20556=ORIENTED_EDGE('',*,*,#14996,.T.);
#20557=ORIENTED_EDGE('',*,*,#14997,.F.);
#20558=ORIENTED_EDGE('',*,*,#14969,.F.);
#20559=ORIENTED_EDGE('',*,*,#14995,.T.);
#20560=ORIENTED_EDGE('',*,*,#14941,.F.);
#20561=ORIENTED_EDGE('',*,*,#14953,.F.);
#20562=ORIENTED_EDGE('',*,*,#14998,.T.);
#20563=ORIENTED_EDGE('',*,*,#14999,.F.);
#20564=ORIENTED_EDGE('',*,*,#14970,.F.);
#20565=ORIENTED_EDGE('',*,*,#14997,.T.);
#20566=ORIENTED_EDGE('',*,*,#15000,.T.);
#20567=ORIENTED_EDGE('',*,*,#15001,.F.);
#20568=ORIENTED_EDGE('',*,*,#14971,.F.);
#20569=ORIENTED_EDGE('',*,*,#14999,.T.);
#20570=ORIENTED_EDGE('',*,*,#15002,.T.);
#20571=ORIENTED_EDGE('',*,*,#15003,.F.);
#20572=ORIENTED_EDGE('',*,*,#14972,.F.);
#20573=ORIENTED_EDGE('',*,*,#15001,.T.);
#20574=ORIENTED_EDGE('',*,*,#15004,.T.);
#20575=ORIENTED_EDGE('',*,*,#15005,.F.);
#20576=ORIENTED_EDGE('',*,*,#14973,.F.);
#20577=ORIENTED_EDGE('',*,*,#15003,.T.);
#20578=ORIENTED_EDGE('',*,*,#15006,.T.);
#20579=ORIENTED_EDGE('',*,*,#14985,.F.);
#20580=ORIENTED_EDGE('',*,*,#14974,.F.);
#20581=ORIENTED_EDGE('',*,*,#15005,.T.);
#20582=ORIENTED_EDGE('',*,*,#14983,.F.);
#20583=ORIENTED_EDGE('',*,*,#15006,.F.);
#20584=ORIENTED_EDGE('',*,*,#15004,.F.);
#20585=ORIENTED_EDGE('',*,*,#15002,.F.);
#20586=ORIENTED_EDGE('',*,*,#15000,.F.);
#20587=ORIENTED_EDGE('',*,*,#14998,.F.);
#20588=ORIENTED_EDGE('',*,*,#14996,.F.);
#20589=ORIENTED_EDGE('',*,*,#14994,.F.);
#20590=ORIENTED_EDGE('',*,*,#14992,.F.);
#20591=ORIENTED_EDGE('',*,*,#14990,.F.);
#20592=ORIENTED_EDGE('',*,*,#14988,.F.);
#20593=ORIENTED_EDGE('',*,*,#14986,.F.);
#20594=ORIENTED_EDGE('',*,*,#14912,.T.);
#20595=ORIENTED_EDGE('',*,*,#14957,.T.);
#20596=ORIENTED_EDGE('',*,*,#14962,.F.);
#20597=ORIENTED_EDGE('',*,*,#14951,.T.);
#20598=ORIENTED_EDGE('',*,*,#14956,.F.);
#20599=ORIENTED_EDGE('',*,*,#14945,.T.);
#20600=ORIENTED_EDGE('',*,*,#14950,.F.);
#20601=ORIENTED_EDGE('',*,*,#14939,.T.);
#20602=ORIENTED_EDGE('',*,*,#14944,.F.);
#20603=ORIENTED_EDGE('',*,*,#15007,.T.);
#20604=ORIENTED_EDGE('',*,*,#15008,.T.);
#20605=ORIENTED_EDGE('',*,*,#15009,.T.);
#20606=ORIENTED_EDGE('',*,*,#15010,.T.);
#20607=ORIENTED_EDGE('',*,*,#15011,.T.);
#20608=ORIENTED_EDGE('',*,*,#15012,.T.);
#20609=ORIENTED_EDGE('',*,*,#15013,.T.);
#20610=ORIENTED_EDGE('',*,*,#15014,.T.);
#20611=ORIENTED_EDGE('',*,*,#14936,.F.);
#20612=ORIENTED_EDGE('',*,*,#14933,.F.);
#20613=ORIENTED_EDGE('',*,*,#14930,.F.);
#20614=ORIENTED_EDGE('',*,*,#14927,.F.);
#20615=ORIENTED_EDGE('',*,*,#14902,.F.);
#20616=ORIENTED_EDGE('',*,*,#14976,.T.);
#20617=ORIENTED_EDGE('',*,*,#15015,.F.);
#20618=ORIENTED_EDGE('',*,*,#15007,.F.);
#20619=ORIENTED_EDGE('',*,*,#15016,.T.);
#20620=ORIENTED_EDGE('',*,*,#14975,.T.);
#20621=ORIENTED_EDGE('',*,*,#15017,.F.);
#20622=ORIENTED_EDGE('',*,*,#15008,.F.);
#20623=ORIENTED_EDGE('',*,*,#15015,.T.);
#20624=ORIENTED_EDGE('',*,*,#14982,.T.);
#20625=ORIENTED_EDGE('',*,*,#15018,.F.);
#20626=ORIENTED_EDGE('',*,*,#15009,.F.);
#20627=ORIENTED_EDGE('',*,*,#15017,.T.);
#20628=ORIENTED_EDGE('',*,*,#14981,.T.);
#20629=ORIENTED_EDGE('',*,*,#15019,.F.);
#20630=ORIENTED_EDGE('',*,*,#15010,.F.);
#20631=ORIENTED_EDGE('',*,*,#15018,.T.);
#20632=ORIENTED_EDGE('',*,*,#14980,.T.);
#20633=ORIENTED_EDGE('',*,*,#15020,.F.);
#20634=ORIENTED_EDGE('',*,*,#15011,.F.);
#20635=ORIENTED_EDGE('',*,*,#15019,.T.);
#20636=ORIENTED_EDGE('',*,*,#14979,.T.);
#20637=ORIENTED_EDGE('',*,*,#15021,.F.);
#20638=ORIENTED_EDGE('',*,*,#15012,.F.);
#20639=ORIENTED_EDGE('',*,*,#15020,.T.);
#20640=ORIENTED_EDGE('',*,*,#14978,.T.);
#20641=ORIENTED_EDGE('',*,*,#15022,.F.);
#20642=ORIENTED_EDGE('',*,*,#15013,.F.);
#20643=ORIENTED_EDGE('',*,*,#15021,.T.);
#20644=ORIENTED_EDGE('',*,*,#14977,.T.);
#20645=ORIENTED_EDGE('',*,*,#15016,.F.);
#20646=ORIENTED_EDGE('',*,*,#15014,.F.);
#20647=ORIENTED_EDGE('',*,*,#15022,.T.);
#20648=ORIENTED_EDGE('',*,*,#14926,.T.);
#20649=ORIENTED_EDGE('',*,*,#15023,.F.);
#20650=ORIENTED_EDGE('',*,*,#15024,.F.);
#20651=ORIENTED_EDGE('',*,*,#15025,.F.);
#20652=ORIENTED_EDGE('',*,*,#15026,.F.);
#20653=ORIENTED_EDGE('',*,*,#15027,.F.);
#20654=ORIENTED_EDGE('',*,*,#15028,.F.);
#20655=ORIENTED_EDGE('',*,*,#14923,.T.);
#20656=ORIENTED_EDGE('',*,*,#15029,.F.);
#20657=ORIENTED_EDGE('',*,*,#15030,.F.);
#20658=ORIENTED_EDGE('',*,*,#15031,.F.);
#20659=ORIENTED_EDGE('',*,*,#15032,.F.);
#20660=ORIENTED_EDGE('',*,*,#15033,.F.);
#20661=ORIENTED_EDGE('',*,*,#15034,.F.);
#20662=ORIENTED_EDGE('',*,*,#14920,.T.);
#20663=ORIENTED_EDGE('',*,*,#15035,.F.);
#20664=ORIENTED_EDGE('',*,*,#15036,.F.);
#20665=ORIENTED_EDGE('',*,*,#15037,.F.);
#20666=ORIENTED_EDGE('',*,*,#15038,.F.);
#20667=ORIENTED_EDGE('',*,*,#15039,.F.);
#20668=ORIENTED_EDGE('',*,*,#15040,.F.);
#20669=ORIENTED_EDGE('',*,*,#14917,.T.);
#20670=ORIENTED_EDGE('',*,*,#15041,.F.);
#20671=ORIENTED_EDGE('',*,*,#15042,.F.);
#20672=ORIENTED_EDGE('',*,*,#15043,.F.);
#20673=ORIENTED_EDGE('',*,*,#15044,.F.);
#20674=ORIENTED_EDGE('',*,*,#15045,.F.);
#20675=ORIENTED_EDGE('',*,*,#15046,.F.);
#20676=ORIENTED_EDGE('',*,*,#15023,.T.);
#20677=ORIENTED_EDGE('',*,*,#15047,.F.);
#20678=ORIENTED_EDGE('',*,*,#15048,.F.);
#20679=ORIENTED_EDGE('',*,*,#15049,.T.);
#20680=ORIENTED_EDGE('',*,*,#15024,.T.);
#20681=ORIENTED_EDGE('',*,*,#15049,.F.);
#20682=ORIENTED_EDGE('',*,*,#15050,.F.);
#20683=ORIENTED_EDGE('',*,*,#15051,.T.);
#20684=ORIENTED_EDGE('',*,*,#15025,.T.);
#20685=ORIENTED_EDGE('',*,*,#15051,.F.);
#20686=ORIENTED_EDGE('',*,*,#15052,.F.);
#20687=ORIENTED_EDGE('',*,*,#15053,.T.);
#20688=ORIENTED_EDGE('',*,*,#15026,.T.);
#20689=ORIENTED_EDGE('',*,*,#15053,.F.);
#20690=ORIENTED_EDGE('',*,*,#15054,.F.);
#20691=ORIENTED_EDGE('',*,*,#15055,.T.);
#20692=ORIENTED_EDGE('',*,*,#15027,.T.);
#20693=ORIENTED_EDGE('',*,*,#15055,.F.);
#20694=ORIENTED_EDGE('',*,*,#15056,.F.);
#20695=ORIENTED_EDGE('',*,*,#15057,.T.);
#20696=ORIENTED_EDGE('',*,*,#15028,.T.);
#20697=ORIENTED_EDGE('',*,*,#15057,.F.);
#20698=ORIENTED_EDGE('',*,*,#15058,.F.);
#20699=ORIENTED_EDGE('',*,*,#15047,.T.);
#20700=ORIENTED_EDGE('',*,*,#15048,.T.);
#20701=ORIENTED_EDGE('',*,*,#15058,.T.);
#20702=ORIENTED_EDGE('',*,*,#15056,.T.);
#20703=ORIENTED_EDGE('',*,*,#15054,.T.);
#20704=ORIENTED_EDGE('',*,*,#15052,.T.);
#20705=ORIENTED_EDGE('',*,*,#15050,.T.);
#20706=ORIENTED_EDGE('',*,*,#15029,.T.);
#20707=ORIENTED_EDGE('',*,*,#15059,.F.);
#20708=ORIENTED_EDGE('',*,*,#15060,.F.);
#20709=ORIENTED_EDGE('',*,*,#15061,.T.);
#20710=ORIENTED_EDGE('',*,*,#15030,.T.);
#20711=ORIENTED_EDGE('',*,*,#15061,.F.);
#20712=ORIENTED_EDGE('',*,*,#15062,.F.);
#20713=ORIENTED_EDGE('',*,*,#15063,.T.);
#20714=ORIENTED_EDGE('',*,*,#15031,.T.);
#20715=ORIENTED_EDGE('',*,*,#15063,.F.);
#20716=ORIENTED_EDGE('',*,*,#15064,.F.);
#20717=ORIENTED_EDGE('',*,*,#15065,.T.);
#20718=ORIENTED_EDGE('',*,*,#15032,.T.);
#20719=ORIENTED_EDGE('',*,*,#15065,.F.);
#20720=ORIENTED_EDGE('',*,*,#15066,.F.);
#20721=ORIENTED_EDGE('',*,*,#15067,.T.);
#20722=ORIENTED_EDGE('',*,*,#15033,.T.);
#20723=ORIENTED_EDGE('',*,*,#15067,.F.);
#20724=ORIENTED_EDGE('',*,*,#15068,.F.);
#20725=ORIENTED_EDGE('',*,*,#15069,.T.);
#20726=ORIENTED_EDGE('',*,*,#15034,.T.);
#20727=ORIENTED_EDGE('',*,*,#15069,.F.);
#20728=ORIENTED_EDGE('',*,*,#15070,.F.);
#20729=ORIENTED_EDGE('',*,*,#15059,.T.);
#20730=ORIENTED_EDGE('',*,*,#15060,.T.);
#20731=ORIENTED_EDGE('',*,*,#15070,.T.);
#20732=ORIENTED_EDGE('',*,*,#15068,.T.);
#20733=ORIENTED_EDGE('',*,*,#15066,.T.);
#20734=ORIENTED_EDGE('',*,*,#15064,.T.);
#20735=ORIENTED_EDGE('',*,*,#15062,.T.);
#20736=ORIENTED_EDGE('',*,*,#15041,.T.);
#20737=ORIENTED_EDGE('',*,*,#15071,.F.);
#20738=ORIENTED_EDGE('',*,*,#15072,.F.);
#20739=ORIENTED_EDGE('',*,*,#15073,.T.);
#20740=ORIENTED_EDGE('',*,*,#15042,.T.);
#20741=ORIENTED_EDGE('',*,*,#15073,.F.);
#20742=ORIENTED_EDGE('',*,*,#15074,.F.);
#20743=ORIENTED_EDGE('',*,*,#15075,.T.);
#20744=ORIENTED_EDGE('',*,*,#15043,.T.);
#20745=ORIENTED_EDGE('',*,*,#15075,.F.);
#20746=ORIENTED_EDGE('',*,*,#15076,.F.);
#20747=ORIENTED_EDGE('',*,*,#15077,.T.);
#20748=ORIENTED_EDGE('',*,*,#15044,.T.);
#20749=ORIENTED_EDGE('',*,*,#15077,.F.);
#20750=ORIENTED_EDGE('',*,*,#15078,.F.);
#20751=ORIENTED_EDGE('',*,*,#15079,.T.);
#20752=ORIENTED_EDGE('',*,*,#15045,.T.);
#20753=ORIENTED_EDGE('',*,*,#15079,.F.);
#20754=ORIENTED_EDGE('',*,*,#15080,.F.);
#20755=ORIENTED_EDGE('',*,*,#15081,.T.);
#20756=ORIENTED_EDGE('',*,*,#15046,.T.);
#20757=ORIENTED_EDGE('',*,*,#15081,.F.);
#20758=ORIENTED_EDGE('',*,*,#15082,.F.);
#20759=ORIENTED_EDGE('',*,*,#15071,.T.);
#20760=ORIENTED_EDGE('',*,*,#15072,.T.);
#20761=ORIENTED_EDGE('',*,*,#15082,.T.);
#20762=ORIENTED_EDGE('',*,*,#15080,.T.);
#20763=ORIENTED_EDGE('',*,*,#15078,.T.);
#20764=ORIENTED_EDGE('',*,*,#15076,.T.);
#20765=ORIENTED_EDGE('',*,*,#15074,.T.);
#20766=ORIENTED_EDGE('',*,*,#15035,.T.);
#20767=ORIENTED_EDGE('',*,*,#15083,.F.);
#20768=ORIENTED_EDGE('',*,*,#15084,.F.);
#20769=ORIENTED_EDGE('',*,*,#15085,.T.);
#20770=ORIENTED_EDGE('',*,*,#15036,.T.);
#20771=ORIENTED_EDGE('',*,*,#15085,.F.);
#20772=ORIENTED_EDGE('',*,*,#15086,.F.);
#20773=ORIENTED_EDGE('',*,*,#15087,.T.);
#20774=ORIENTED_EDGE('',*,*,#15037,.T.);
#20775=ORIENTED_EDGE('',*,*,#15087,.F.);
#20776=ORIENTED_EDGE('',*,*,#15088,.F.);
#20777=ORIENTED_EDGE('',*,*,#15089,.T.);
#20778=ORIENTED_EDGE('',*,*,#15038,.T.);
#20779=ORIENTED_EDGE('',*,*,#15089,.F.);
#20780=ORIENTED_EDGE('',*,*,#15090,.F.);
#20781=ORIENTED_EDGE('',*,*,#15091,.T.);
#20782=ORIENTED_EDGE('',*,*,#15039,.T.);
#20783=ORIENTED_EDGE('',*,*,#15091,.F.);
#20784=ORIENTED_EDGE('',*,*,#15092,.F.);
#20785=ORIENTED_EDGE('',*,*,#15093,.T.);
#20786=ORIENTED_EDGE('',*,*,#15040,.T.);
#20787=ORIENTED_EDGE('',*,*,#15093,.F.);
#20788=ORIENTED_EDGE('',*,*,#15094,.F.);
#20789=ORIENTED_EDGE('',*,*,#15083,.T.);
#20790=ORIENTED_EDGE('',*,*,#15084,.T.);
#20791=ORIENTED_EDGE('',*,*,#15094,.T.);
#20792=ORIENTED_EDGE('',*,*,#15092,.T.);
#20793=ORIENTED_EDGE('',*,*,#15090,.T.);
#20794=ORIENTED_EDGE('',*,*,#15088,.T.);
#20795=ORIENTED_EDGE('',*,*,#15086,.T.);
#20796=ORIENTED_EDGE('',*,*,#14914,.F.);
#20797=ORIENTED_EDGE('',*,*,#14909,.T.);
#20798=ORIENTED_EDGE('',*,*,#14911,.F.);
#20799=ORIENTED_EDGE('',*,*,#14906,.T.);
#20800=ORIENTED_EDGE('',*,*,#14903,.T.);
#20801=ORIENTED_EDGE('',*,*,#14908,.F.);
#20802=ORIENTED_EDGE('',*,*,#14900,.T.);
#20803=ORIENTED_EDGE('',*,*,#14905,.F.);
#24057=CYLINDRICAL_SURFACE('',#27472,14.);
#24058=CYLINDRICAL_SURFACE('',#27475,9.75);
#24059=CYLINDRICAL_SURFACE('',#27478,7.5);
#24060=CYLINDRICAL_SURFACE('',#27481,9.75);
#24061=CYLINDRICAL_SURFACE('',#27484,14.);
#24062=CYLINDRICAL_SURFACE('',#27487,3.1);
#24063=CYLINDRICAL_SURFACE('',#27490,3.1);
#24064=CYLINDRICAL_SURFACE('',#27493,3.1);
#24065=CYLINDRICAL_SURFACE('',#27496,3.1);
#24066=CYLINDRICAL_SURFACE('',#27499,3.50000000000001);
#24067=CYLINDRICAL_SURFACE('',#27502,3.5);
#24068=CYLINDRICAL_SURFACE('',#27505,3.50000000000001);
#24069=CYLINDRICAL_SURFACE('',#27508,3.50000000000001);
#24070=CYLINDRICAL_SURFACE('',#27511,5.5);
#24071=CYLINDRICAL_SURFACE('',#27514,3.3);
#24072=CYLINDRICAL_SURFACE('',#27517,5.5);
#24073=CYLINDRICAL_SURFACE('',#27520,3.3);
#24074=CYLINDRICAL_SURFACE('',#27523,5.5);
#24075=CYLINDRICAL_SURFACE('',#27526,3.3);
#24076=CYLINDRICAL_SURFACE('',#27529,5.5);
#24077=CYLINDRICAL_SURFACE('',#27532,3.3);
#24929=ADVANCED_FACE('',(#2976),#24057,.F.);
#24930=ADVANCED_FACE('',(#2977),#24058,.F.);
#24931=ADVANCED_FACE('',(#2978),#24059,.F.);
#24932=ADVANCED_FACE('',(#2979),#24060,.F.);
#24933=ADVANCED_FACE('',(#2980),#24061,.F.);
#24934=ADVANCED_FACE('',(#2981),#24062,.T.);
#24935=ADVANCED_FACE('',(#2982),#24063,.T.);
#24936=ADVANCED_FACE('',(#2983),#24064,.T.);
#24937=ADVANCED_FACE('',(#2984),#24065,.T.);
#24938=ADVANCED_FACE('',(#2985),#24066,.F.);
#24939=ADVANCED_FACE('',(#2986),#24067,.F.);
#24940=ADVANCED_FACE('',(#2987),#24068,.F.);
#24941=ADVANCED_FACE('',(#2988),#24069,.F.);
#24942=ADVANCED_FACE('',(#2989),#24070,.F.);
#24943=ADVANCED_FACE('',(#2990),#24071,.F.);
#24944=ADVANCED_FACE('',(#2991),#24072,.F.);
#24945=ADVANCED_FACE('',(#2992),#24073,.F.);
#24946=ADVANCED_FACE('',(#2993),#24074,.F.);
#24947=ADVANCED_FACE('',(#2994),#24075,.F.);
#24948=ADVANCED_FACE('',(#2995),#24076,.F.);
#24949=ADVANCED_FACE('',(#2996),#24077,.F.);
#24950=ADVANCED_FACE('',(#2997,#1342),#1915,.T.);
#24951=ADVANCED_FACE('',(#2998,#1343),#1916,.T.);
#24952=ADVANCED_FACE('',(#2999,#1344),#1917,.T.);
#24953=ADVANCED_FACE('',(#3000,#1345),#1918,.T.);
#24954=ADVANCED_FACE('',(#3001,#1346),#1919,.T.);
#24955=ADVANCED_FACE('',(#3002,#1347,#1348),#1920,.F.);
#24956=ADVANCED_FACE('',(#3003),#1921,.F.);
#24957=ADVANCED_FACE('',(#3004),#1922,.F.);
#24958=ADVANCED_FACE('',(#3005,#1349,#1350,#1351,#1352),#1923,.F.);
#24959=ADVANCED_FACE('',(#3006),#1924,.F.);
#24960=ADVANCED_FACE('',(#3007),#1925,.F.);
#24961=ADVANCED_FACE('',(#3008,#1353,#1354),#1926,.F.);
#24962=ADVANCED_FACE('',(#3009),#1927,.F.);
#24963=ADVANCED_FACE('',(#3010),#1928,.F.);
#24964=ADVANCED_FACE('',(#3011),#1929,.F.);
#24965=ADVANCED_FACE('',(#3012),#1930,.F.);
#24966=ADVANCED_FACE('',(#3013),#1931,.F.);
#24967=ADVANCED_FACE('',(#3014,#1355),#1932,.F.);
#24968=ADVANCED_FACE('',(#3015,#1356),#1933,.F.);
#24969=ADVANCED_FACE('',(#3016,#1357),#1934,.F.);
#24970=ADVANCED_FACE('',(#3017,#1358),#1935,.F.);
#24971=ADVANCED_FACE('',(#3018,#1359),#1936,.F.);
#24972=ADVANCED_FACE('',(#3019,#1360,#1361,#1362,#1363,#1364),#1937,.F.);
#24973=ADVANCED_FACE('',(#3020),#1938,.F.);
#24974=ADVANCED_FACE('',(#3021),#1939,.F.);
#24975=ADVANCED_FACE('',(#3022),#1940,.F.);
#24976=ADVANCED_FACE('',(#3023),#1941,.F.);
#24977=ADVANCED_FACE('',(#3024),#1942,.F.);
#24978=ADVANCED_FACE('',(#3025),#1943,.F.);
#24979=ADVANCED_FACE('',(#3026),#1944,.F.);
#24980=ADVANCED_FACE('',(#3027),#1945,.F.);
#24981=ADVANCED_FACE('',(#3028,#1365),#1946,.T.);
#24982=ADVANCED_FACE('',(#3029,#1366),#1947,.T.);
#24983=ADVANCED_FACE('',(#3030,#1367),#1948,.T.);
#24984=ADVANCED_FACE('',(#3031,#1368),#1949,.T.);
#24985=ADVANCED_FACE('',(#3032),#1950,.F.);
#24986=ADVANCED_FACE('',(#3033),#1951,.F.);
#24987=ADVANCED_FACE('',(#3034),#1952,.F.);
#24988=ADVANCED_FACE('',(#3035),#1953,.F.);
#24989=ADVANCED_FACE('',(#3036),#1954,.F.);
#24990=ADVANCED_FACE('',(#3037),#1955,.F.);
#24991=ADVANCED_FACE('',(#3038),#1956,.T.);
#24992=ADVANCED_FACE('',(#3039),#1957,.F.);
#24993=ADVANCED_FACE('',(#3040),#1958,.F.);
#24994=ADVANCED_FACE('',(#3041),#1959,.F.);
#24995=ADVANCED_FACE('',(#3042),#1960,.F.);
#24996=ADVANCED_FACE('',(#3043),#1961,.F.);
#24997=ADVANCED_FACE('',(#3044),#1962,.F.);
#24998=ADVANCED_FACE('',(#3045),#1963,.T.);
#24999=ADVANCED_FACE('',(#3046),#1964,.F.);
#25000=ADVANCED_FACE('',(#3047),#1965,.F.);
#25001=ADVANCED_FACE('',(#3048),#1966,.F.);
#25002=ADVANCED_FACE('',(#3049),#1967,.F.);
#25003=ADVANCED_FACE('',(#3050),#1968,.F.);
#25004=ADVANCED_FACE('',(#3051),#1969,.F.);
#25005=ADVANCED_FACE('',(#3052),#1970,.T.);
#25006=ADVANCED_FACE('',(#3053),#1971,.F.);
#25007=ADVANCED_FACE('',(#3054),#1972,.F.);
#25008=ADVANCED_FACE('',(#3055),#1973,.F.);
#25009=ADVANCED_FACE('',(#3056),#1974,.F.);
#25010=ADVANCED_FACE('',(#3057),#1975,.F.);
#25011=ADVANCED_FACE('',(#3058),#1976,.F.);
#25012=ADVANCED_FACE('',(#3059),#1977,.T.);
#25013=ADVANCED_FACE('',(#3060,#1369),#1978,.F.);
#25014=ADVANCED_FACE('',(#3061,#1370),#1979,.F.);
#25015=ADVANCED_FACE('',(#3062,#1371),#1980,.F.);
#25016=ADVANCED_FACE('',(#3063,#1372),#1981,.F.);
#25677=CLOSED_SHELL('',(#24929,#24930,#24931,#24932,#24933,#24934,#24935,
#24936,#24937,#24938,#24939,#24940,#24941,#24942,#24943,#24944,#24945,#24946,
#24947,#24948,#24949,#24950,#24951,#24952,#24953,#24954,#24955,#24956,#24957,
#24958,#24959,#24960,#24961,#24962,#24963,#24964,#24965,#24966,#24967,#24968,
#24969,#24970,#24971,#24972,#24973,#24974,#24975,#24976,#24977,#24978,#24979,
#24980,#24981,#24982,#24983,#24984,#24985,#24986,#24987,#24988,#24989,#24990,
#24991,#24992,#24993,#24994,#24995,#24996,#24997,#24998,#24999,#25000,#25001,
#25002,#25003,#25004,#25005,#25006,#25007,#25008,#25009,#25010,#25011,#25012,
#25013,#25014,#25015,#25016));
#27471=AXIS2_PLACEMENT_3D('',#40424,#32791,#32792);
#27472=AXIS2_PLACEMENT_3D('',#40425,#32793,#32794);
#27473=AXIS2_PLACEMENT_3D('',#40427,#32795,#32796);
#27474=AXIS2_PLACEMENT_3D('',#40430,#32798,#32799);
#27475=AXIS2_PLACEMENT_3D('',#40431,#32800,#32801);
#27476=AXIS2_PLACEMENT_3D('',#40433,#32802,#32803);
#27477=AXIS2_PLACEMENT_3D('',#40436,#32805,#32806);
#27478=AXIS2_PLACEMENT_3D('',#40437,#32807,#32808);
#27479=AXIS2_PLACEMENT_3D('',#40439,#32809,#32810);
#27480=AXIS2_PLACEMENT_3D('',#40442,#32812,#32813);
#27481=AXIS2_PLACEMENT_3D('',#40443,#32814,#32815);
#27482=AXIS2_PLACEMENT_3D('',#40445,#32816,#32817);
#27483=AXIS2_PLACEMENT_3D('',#40448,#32819,#32820);
#27484=AXIS2_PLACEMENT_3D('',#40449,#32821,#32822);
#27485=AXIS2_PLACEMENT_3D('',#40451,#32823,#32824);
#27486=AXIS2_PLACEMENT_3D('',#40454,#32826,#32827);
#27487=AXIS2_PLACEMENT_3D('',#40455,#32828,#32829);
#27488=AXIS2_PLACEMENT_3D('',#40457,#32830,#32831);
#27489=AXIS2_PLACEMENT_3D('',#40460,#32833,#32834);
#27490=AXIS2_PLACEMENT_3D('',#40461,#32835,#32836);
#27491=AXIS2_PLACEMENT_3D('',#40463,#32837,#32838);
#27492=AXIS2_PLACEMENT_3D('',#40466,#32840,#32841);
#27493=AXIS2_PLACEMENT_3D('',#40467,#32842,#32843);
#27494=AXIS2_PLACEMENT_3D('',#40469,#32844,#32845);
#27495=AXIS2_PLACEMENT_3D('',#40472,#32847,#32848);
#27496=AXIS2_PLACEMENT_3D('',#40473,#32849,#32850);
#27497=AXIS2_PLACEMENT_3D('',#40475,#32851,#32852);
#27498=AXIS2_PLACEMENT_3D('',#40478,#32854,#32855);
#27499=AXIS2_PLACEMENT_3D('',#40479,#32856,#32857);
#27500=AXIS2_PLACEMENT_3D('',#40481,#32858,#32859);
#27501=AXIS2_PLACEMENT_3D('',#40484,#32861,#32862);
#27502=AXIS2_PLACEMENT_3D('',#40485,#32863,#32864);
#27503=AXIS2_PLACEMENT_3D('',#40487,#32865,#32866);
#27504=AXIS2_PLACEMENT_3D('',#40490,#32868,#32869);
#27505=AXIS2_PLACEMENT_3D('',#40491,#32870,#32871);
#27506=AXIS2_PLACEMENT_3D('',#40493,#32872,#32873);
#27507=AXIS2_PLACEMENT_3D('',#40496,#32875,#32876);
#27508=AXIS2_PLACEMENT_3D('',#40497,#32877,#32878);
#27509=AXIS2_PLACEMENT_3D('',#40499,#32879,#32880);
#27510=AXIS2_PLACEMENT_3D('',#40502,#32882,#32883);
#27511=AXIS2_PLACEMENT_3D('',#40503,#32884,#32885);
#27512=AXIS2_PLACEMENT_3D('',#40505,#32886,#32887);
#27513=AXIS2_PLACEMENT_3D('',#40508,#32889,#32890);
#27514=AXIS2_PLACEMENT_3D('',#40509,#32891,#32892);
#27515=AXIS2_PLACEMENT_3D('',#40511,#32893,#32894);
#27516=AXIS2_PLACEMENT_3D('',#40514,#32896,#32897);
#27517=AXIS2_PLACEMENT_3D('',#40515,#32898,#32899);
#27518=AXIS2_PLACEMENT_3D('',#40517,#32900,#32901);
#27519=AXIS2_PLACEMENT_3D('',#40520,#32903,#32904);
#27520=AXIS2_PLACEMENT_3D('',#40521,#32905,#32906);
#27521=AXIS2_PLACEMENT_3D('',#40523,#32907,#32908);
#27522=AXIS2_PLACEMENT_3D('',#40526,#32910,#32911);
#27523=AXIS2_PLACEMENT_3D('',#40527,#32912,#32913);
#27524=AXIS2_PLACEMENT_3D('',#40529,#32914,#32915);
#27525=AXIS2_PLACEMENT_3D('',#40532,#32917,#32918);
#27526=AXIS2_PLACEMENT_3D('',#40533,#32919,#32920);
#27527=AXIS2_PLACEMENT_3D('',#40535,#32921,#32922);
#27528=AXIS2_PLACEMENT_3D('',#40538,#32924,#32925);
#27529=AXIS2_PLACEMENT_3D('',#40539,#32926,#32927);
#27530=AXIS2_PLACEMENT_3D('',#40541,#32928,#32929);
#27531=AXIS2_PLACEMENT_3D('',#40544,#32931,#32932);
#27532=AXIS2_PLACEMENT_3D('',#40545,#32933,#32934);
#27533=AXIS2_PLACEMENT_3D('',#40547,#32935,#32936);
#27534=AXIS2_PLACEMENT_3D('',#40550,#32938,#32939);
#27535=AXIS2_PLACEMENT_3D('',#40551,#32940,#32941);
#27536=AXIS2_PLACEMENT_3D('',#40552,#32942,#32943);
#27537=AXIS2_PLACEMENT_3D('',#40553,#32944,#32945);
#27538=AXIS2_PLACEMENT_3D('',#40554,#32946,#32947);
#27539=AXIS2_PLACEMENT_3D('',#40555,#32948,#32949);
#27540=AXIS2_PLACEMENT_3D('',#40596,#32970,#32971);
#27541=AXIS2_PLACEMENT_3D('',#40602,#32975,#32976);
#27542=AXIS2_PLACEMENT_3D('',#40606,#32979,#32980);
#27543=AXIS2_PLACEMENT_3D('',#40610,#32983,#32984);
#27544=AXIS2_PLACEMENT_3D('',#40614,#32987,#32988);
#27545=AXIS2_PLACEMENT_3D('',#40618,#32991,#32992);
#27546=AXIS2_PLACEMENT_3D('',#40622,#32995,#32996);
#27547=AXIS2_PLACEMENT_3D('',#40626,#32999,#33000);
#27548=AXIS2_PLACEMENT_3D('',#40630,#33003,#33004);
#27549=AXIS2_PLACEMENT_3D('',#40634,#33007,#33008);
#27550=AXIS2_PLACEMENT_3D('',#40638,#33011,#33012);
#27551=AXIS2_PLACEMENT_3D('',#40642,#33015,#33016);
#27552=AXIS2_PLACEMENT_3D('',#40644,#33018,#33019);
#27553=AXIS2_PLACEMENT_3D('',#40645,#33020,#33021);
#27554=AXIS2_PLACEMENT_3D('',#40646,#33022,#33023);
#27555=AXIS2_PLACEMENT_3D('',#40647,#33024,#33025);
#27556=AXIS2_PLACEMENT_3D('',#40648,#33026,#33027);
#27557=AXIS2_PLACEMENT_3D('',#40649,#33028,#33029);
#27558=AXIS2_PLACEMENT_3D('',#40666,#33038,#33039);
#27559=AXIS2_PLACEMENT_3D('',#40669,#33042,#33043);
#27560=AXIS2_PLACEMENT_3D('',#40671,#33045,#33046);
#27561=AXIS2_PLACEMENT_3D('',#40673,#33048,#33049);
#27562=AXIS2_PLACEMENT_3D('',#40675,#33051,#33052);
#27563=AXIS2_PLACEMENT_3D('',#40677,#33054,#33055);
#27564=AXIS2_PLACEMENT_3D('',#40679,#33057,#33058);
#27565=AXIS2_PLACEMENT_3D('',#40681,#33060,#33061);
#27566=AXIS2_PLACEMENT_3D('',#40682,#33062,#33063);
#27567=AXIS2_PLACEMENT_3D('',#40695,#33070,#33071);
#27568=AXIS2_PLACEMENT_3D('',#40708,#33078,#33079);
#27569=AXIS2_PLACEMENT_3D('',#40721,#33086,#33087);
#27570=AXIS2_PLACEMENT_3D('',#40734,#33094,#33095);
#27571=AXIS2_PLACEMENT_3D('',#40740,#33099,#33100);
#27572=AXIS2_PLACEMENT_3D('',#40744,#33103,#33104);
#27573=AXIS2_PLACEMENT_3D('',#40748,#33107,#33108);
#27574=AXIS2_PLACEMENT_3D('',#40752,#33111,#33112);
#27575=AXIS2_PLACEMENT_3D('',#40756,#33115,#33116);
#27576=AXIS2_PLACEMENT_3D('',#40758,#33118,#33119);
#27577=AXIS2_PLACEMENT_3D('',#40759,#33120,#33121);
#27578=AXIS2_PLACEMENT_3D('',#40765,#33125,#33126);
#27579=AXIS2_PLACEMENT_3D('',#40769,#33129,#33130);
#27580=AXIS2_PLACEMENT_3D('',#40773,#33133,#33134);
#27581=AXIS2_PLACEMENT_3D('',#40777,#33137,#33138);
#27582=AXIS2_PLACEMENT_3D('',#40781,#33141,#33142);
#27583=AXIS2_PLACEMENT_3D('',#40783,#33144,#33145);
#27584=AXIS2_PLACEMENT_3D('',#40784,#33146,#33147);
#27585=AXIS2_PLACEMENT_3D('',#40790,#33151,#33152);
#27586=AXIS2_PLACEMENT_3D('',#40794,#33155,#33156);
#27587=AXIS2_PLACEMENT_3D('',#40798,#33159,#33160);
#27588=AXIS2_PLACEMENT_3D('',#40802,#33163,#33164);
#27589=AXIS2_PLACEMENT_3D('',#40806,#33167,#33168);
#27590=AXIS2_PLACEMENT_3D('',#40808,#33170,#33171);
#27591=AXIS2_PLACEMENT_3D('',#40809,#33172,#33173);
#27592=AXIS2_PLACEMENT_3D('',#40815,#33177,#33178);
#27593=AXIS2_PLACEMENT_3D('',#40819,#33181,#33182);
#27594=AXIS2_PLACEMENT_3D('',#40823,#33185,#33186);
#27595=AXIS2_PLACEMENT_3D('',#40827,#33189,#33190);
#27596=AXIS2_PLACEMENT_3D('',#40831,#33193,#33194);
#27597=AXIS2_PLACEMENT_3D('',#40833,#33196,#33197);
#27598=AXIS2_PLACEMENT_3D('',#40834,#33198,#33199);
#27599=AXIS2_PLACEMENT_3D('',#40835,#33200,#33201);
#27600=AXIS2_PLACEMENT_3D('',#40836,#33202,#33203);
#27601=AXIS2_PLACEMENT_3D('',#40837,#33204,#33205);
#32791=DIRECTION('axis',(0.,0.,1.));
#32792=DIRECTION('refdir',(1.,0.,0.));
#32793=DIRECTION('center_axis',(1.,0.,0.));
#32794=DIRECTION('ref_axis',(0.,0.,-1.));
#32795=DIRECTION('center_axis',(1.,0.,0.));
#32796=DIRECTION('ref_axis',(0.,0.,-1.));
#32797=DIRECTION('',(1.,0.,0.));
#32798=DIRECTION('center_axis',(1.,0.,0.));
#32799=DIRECTION('ref_axis',(0.,0.,-1.));
#32800=DIRECTION('center_axis',(1.,0.,0.));
#32801=DIRECTION('ref_axis',(0.,0.,-1.));
#32802=DIRECTION('center_axis',(1.,0.,0.));
#32803=DIRECTION('ref_axis',(0.,0.,-1.));
#32804=DIRECTION('',(1.,0.,0.));
#32805=DIRECTION('center_axis',(1.,0.,0.));
#32806=DIRECTION('ref_axis',(0.,0.,-1.));
#32807=DIRECTION('center_axis',(1.,0.,0.));
#32808=DIRECTION('ref_axis',(0.,0.,-1.));
#32809=DIRECTION('center_axis',(1.,0.,0.));
#32810=DIRECTION('ref_axis',(0.,0.,-1.));
#32811=DIRECTION('',(1.,0.,0.));
#32812=DIRECTION('center_axis',(1.,0.,0.));
#32813=DIRECTION('ref_axis',(0.,0.,-1.));
#32814=DIRECTION('center_axis',(1.,0.,0.));
#32815=DIRECTION('ref_axis',(0.,0.,-1.));
#32816=DIRECTION('center_axis',(1.,0.,0.));
#32817=DIRECTION('ref_axis',(0.,0.,-1.));
#32818=DIRECTION('',(1.,0.,0.));
#32819=DIRECTION('center_axis',(1.,0.,0.));
#32820=DIRECTION('ref_axis',(0.,0.,-1.));
#32821=DIRECTION('center_axis',(1.,0.,0.));
#32822=DIRECTION('ref_axis',(0.,0.,-1.));
#32823=DIRECTION('center_axis',(1.,0.,0.));
#32824=DIRECTION('ref_axis',(0.,0.,-1.));
#32825=DIRECTION('',(1.,0.,0.));
#32826=DIRECTION('center_axis',(1.,0.,0.));
#32827=DIRECTION('ref_axis',(0.,0.,-1.));
#32828=DIRECTION('center_axis',(-1.,0.,0.));
#32829=DIRECTION('ref_axis',(0.,0.,1.));
#32830=DIRECTION('center_axis',(1.,0.,0.));
#32831=DIRECTION('ref_axis',(0.,0.,-1.));
#32832=DIRECTION('',(1.,0.,0.));
#32833=DIRECTION('center_axis',(1.,0.,0.));
#32834=DIRECTION('ref_axis',(0.,0.,-1.));
#32835=DIRECTION('center_axis',(-1.,0.,0.));
#32836=DIRECTION('ref_axis',(0.,0.,1.));
#32837=DIRECTION('center_axis',(1.,0.,0.));
#32838=DIRECTION('ref_axis',(0.,0.,-1.));
#32839=DIRECTION('',(1.,0.,0.));
#32840=DIRECTION('center_axis',(1.,0.,0.));
#32841=DIRECTION('ref_axis',(0.,0.,-1.));
#32842=DIRECTION('center_axis',(-1.,0.,0.));
#32843=DIRECTION('ref_axis',(0.,0.,1.));
#32844=DIRECTION('center_axis',(1.,0.,0.));
#32845=DIRECTION('ref_axis',(0.,0.,-1.));
#32846=DIRECTION('',(1.,0.,0.));
#32847=DIRECTION('center_axis',(1.,0.,0.));
#32848=DIRECTION('ref_axis',(0.,0.,-1.));
#32849=DIRECTION('center_axis',(-1.,0.,0.));
#32850=DIRECTION('ref_axis',(0.,0.,1.));
#32851=DIRECTION('center_axis',(1.,0.,0.));
#32852=DIRECTION('ref_axis',(0.,0.,-1.));
#32853=DIRECTION('',(1.,0.,0.));
#32854=DIRECTION('center_axis',(1.,0.,0.));
#32855=DIRECTION('ref_axis',(0.,0.,-1.));
#32856=DIRECTION('center_axis',(-1.,0.,0.));
#32857=DIRECTION('ref_axis',(0.,0.,1.));
#32858=DIRECTION('center_axis',(1.,0.,0.));
#32859=DIRECTION('ref_axis',(0.,0.,-1.));
#32860=DIRECTION('',(-1.,0.,0.));
#32861=DIRECTION('center_axis',(-1.,0.,0.));
#32862=DIRECTION('ref_axis',(0.,0.,-1.));
#32863=DIRECTION('center_axis',(-1.,0.,0.));
#32864=DIRECTION('ref_axis',(0.,0.,1.));
#32865=DIRECTION('center_axis',(1.,0.,0.));
#32866=DIRECTION('ref_axis',(0.,0.,-1.));
#32867=DIRECTION('',(-1.,0.,0.));
#32868=DIRECTION('center_axis',(-1.,0.,0.));
#32869=DIRECTION('ref_axis',(0.,0.,-1.));
#32870=DIRECTION('center_axis',(-1.,0.,0.));
#32871=DIRECTION('ref_axis',(0.,0.,1.));
#32872=DIRECTION('center_axis',(1.,0.,0.));
#32873=DIRECTION('ref_axis',(0.,0.,-1.));
#32874=DIRECTION('',(-1.,0.,0.));
#32875=DIRECTION('center_axis',(-1.,0.,0.));
#32876=DIRECTION('ref_axis',(0.,0.,-1.));
#32877=DIRECTION('center_axis',(-1.,0.,0.));
#32878=DIRECTION('ref_axis',(0.,0.,1.));
#32879=DIRECTION('center_axis',(1.,0.,0.));
#32880=DIRECTION('ref_axis',(0.,0.,-1.));
#32881=DIRECTION('',(-1.,0.,0.));
#32882=DIRECTION('center_axis',(-1.,0.,0.));
#32883=DIRECTION('ref_axis',(0.,0.,-1.));
#32884=DIRECTION('center_axis',(0.,1.,0.));
#32885=DIRECTION('ref_axis',(0.,0.,1.));
#32886=DIRECTION('center_axis',(0.,1.,0.));
#32887=DIRECTION('ref_axis',(0.,0.,1.));
#32888=DIRECTION('',(0.,1.,0.));
#32889=DIRECTION('center_axis',(0.,1.,0.));
#32890=DIRECTION('ref_axis',(0.,0.,1.));
#32891=DIRECTION('center_axis',(0.,1.,0.));
#32892=DIRECTION('ref_axis',(0.,0.,1.));
#32893=DIRECTION('center_axis',(0.,1.,0.));
#32894=DIRECTION('ref_axis',(0.,0.,1.));
#32895=DIRECTION('',(0.,1.,0.));
#32896=DIRECTION('center_axis',(0.,1.,0.));
#32897=DIRECTION('ref_axis',(0.,0.,1.));
#32898=DIRECTION('center_axis',(0.,1.,0.));
#32899=DIRECTION('ref_axis',(0.,0.,1.));
#32900=DIRECTION('center_axis',(0.,1.,0.));
#32901=DIRECTION('ref_axis',(0.,0.,1.));
#32902=DIRECTION('',(0.,1.,0.));
#32903=DIRECTION('center_axis',(0.,1.,0.));
#32904=DIRECTION('ref_axis',(0.,0.,1.));
#32905=DIRECTION('center_axis',(0.,1.,0.));
#32906=DIRECTION('ref_axis',(0.,0.,1.));
#32907=DIRECTION('center_axis',(0.,1.,0.));
#32908=DIRECTION('ref_axis',(0.,0.,1.));
#32909=DIRECTION('',(0.,1.,0.));
#32910=DIRECTION('center_axis',(0.,1.,0.));
#32911=DIRECTION('ref_axis',(0.,0.,1.));
#32912=DIRECTION('center_axis',(0.,1.,0.));
#32913=DIRECTION('ref_axis',(0.,0.,1.));
#32914=DIRECTION('center_axis',(0.,1.,0.));
#32915=DIRECTION('ref_axis',(0.,0.,1.));
#32916=DIRECTION('',(0.,1.,0.));
#32917=DIRECTION('center_axis',(0.,1.,0.));
#32918=DIRECTION('ref_axis',(0.,0.,1.));
#32919=DIRECTION('center_axis',(0.,1.,0.));
#32920=DIRECTION('ref_axis',(0.,0.,1.));
#32921=DIRECTION('center_axis',(0.,1.,0.));
#32922=DIRECTION('ref_axis',(0.,0.,1.));
#32923=DIRECTION('',(0.,1.,0.));
#32924=DIRECTION('center_axis',(0.,1.,0.));
#32925=DIRECTION('ref_axis',(0.,0.,1.));
#32926=DIRECTION('center_axis',(0.,1.,0.));
#32927=DIRECTION('ref_axis',(0.,0.,1.));
#32928=DIRECTION('center_axis',(0.,1.,0.));
#32929=DIRECTION('ref_axis',(0.,0.,1.));
#32930=DIRECTION('',(0.,1.,0.));
#32931=DIRECTION('center_axis',(0.,1.,0.));
#32932=DIRECTION('ref_axis',(0.,0.,1.));
#32933=DIRECTION('center_axis',(0.,1.,0.));
#32934=DIRECTION('ref_axis',(0.,0.,1.));
#32935=DIRECTION('center_axis',(0.,1.,0.));
#32936=DIRECTION('ref_axis',(0.,0.,1.));
#32937=DIRECTION('',(0.,1.,0.));
#32938=DIRECTION('center_axis',(0.,1.,0.));
#32939=DIRECTION('ref_axis',(0.,0.,1.));
#32940=DIRECTION('center_axis',(1.,0.,0.));
#32941=DIRECTION('ref_axis',(0.,0.,-1.));
#32942=DIRECTION('center_axis',(1.,0.,0.));
#32943=DIRECTION('ref_axis',(0.,0.,-1.));
#32944=DIRECTION('center_axis',(1.,0.,0.));
#32945=DIRECTION('ref_axis',(0.,0.,-1.));
#32946=DIRECTION('center_axis',(1.,0.,0.));
#32947=DIRECTION('ref_axis',(0.,0.,-1.));
#32948=DIRECTION('center_axis',(1.,0.,0.));
#32949=DIRECTION('ref_axis',(0.,0.,-1.));
#32950=DIRECTION('',(0.,-4.78544407166016E-16,1.));
#32951=DIRECTION('',(0.,-0.707106781186562,0.707106781186533));
#32952=DIRECTION('',(0.,-1.,-3.70074341541719E-16));
#32953=DIRECTION('',(0.,2.19514413070285E-16,-1.));
#32954=DIRECTION('',(0.,1.,1.8503717077086E-16));
#32955=DIRECTION('',(0.,0.707106781186552,0.707106781186543));
#32956=DIRECTION('',(0.,-4.78544407166016E-16,1.));
#32957=DIRECTION('',(0.,1.,7.30409884621814E-16));
#32958=DIRECTION('',(0.,0.707106781186547,0.707106781186547));
#32959=DIRECTION('',(0.,1.77920356510442E-16,1.));
#32960=DIRECTION('',(0.,-0.707106781186543,0.707106781186552));
#32961=DIRECTION('',(0.,-1.,-7.30409884621814E-16));
#32962=DIRECTION('',(0.,-0.707106781186549,0.707106781186546));
#32963=DIRECTION('',(0.,0.,1.));
#32964=DIRECTION('',(0.,0.707106781186546,0.707106781186549));
#32965=DIRECTION('',(0.,1.,0.));
#32966=DIRECTION('',(0.,0.707106781186549,-0.707106781186546));
#32967=DIRECTION('',(0.,0.,-1.));
#32968=DIRECTION('',(0.,-0.707106781186547,-0.707106781186548));
#32969=DIRECTION('',(0.,-1.,0.));
#32970=DIRECTION('center_axis',(0.,-1.,-4.78544407166016E-16));
#32971=DIRECTION('ref_axis',(0.,4.78544407166016E-16,-1.));
#32972=DIRECTION('',(0.,-4.78544407166016E-16,1.));
#32973=DIRECTION('',(-1.,0.,0.));
#32974=DIRECTION('',(-1.,0.,0.));
#32975=DIRECTION('center_axis',(0.,-0.707106781186533,-0.707106781186562));
#32976=DIRECTION('ref_axis',(0.,0.707106781186562,-0.707106781186533));
#32977=DIRECTION('',(0.,-0.707106781186562,0.707106781186533));
#32978=DIRECTION('',(-1.,0.,0.));
#32979=DIRECTION('center_axis',(0.,3.70074341541719E-16,-1.));
#32980=DIRECTION('ref_axis',(0.,1.,3.70074341541719E-16));
#32981=DIRECTION('',(0.,-1.,-3.70074341541719E-16));
#32982=DIRECTION('',(-1.,0.,0.));
#32983=DIRECTION('center_axis',(0.,1.,2.19514413070285E-16));
#32984=DIRECTION('ref_axis',(0.,-2.19514413070285E-16,1.));
#32985=DIRECTION('',(0.,2.19514413070285E-16,-1.));
#32986=DIRECTION('',(-1.,0.,0.));
#32987=DIRECTION('center_axis',(0.,-1.8503717077086E-16,1.));
#32988=DIRECTION('ref_axis',(0.,-1.,-1.8503717077086E-16));
#32989=DIRECTION('',(0.,1.,1.8503717077086E-16));
#32990=DIRECTION('',(-1.,0.,0.));
#32991=DIRECTION('center_axis',(0.,-0.707106781186543,0.707106781186552));
#32992=DIRECTION('ref_axis',(0.,-0.707106781186553,-0.707106781186543));
#32993=DIRECTION('',(0.,0.707106781186552,0.707106781186543));
#32994=DIRECTION('',(-1.,0.,0.));
#32995=DIRECTION('center_axis',(0.,-1.,-4.78544407166016E-16));
#32996=DIRECTION('ref_axis',(0.,4.78544407166016E-16,-1.));
#32997=DIRECTION('',(0.,-4.78544407166016E-16,1.));
#32998=DIRECTION('',(-1.,0.,0.));
#32999=DIRECTION('center_axis',(0.,-7.30409884621814E-16,1.));
#33000=DIRECTION('ref_axis',(0.,-1.,-7.30409884621815E-16));
#33001=DIRECTION('',(0.,1.,7.30409884621814E-16));
#33002=DIRECTION('',(-1.,0.,0.));
#33003=DIRECTION('center_axis',(0.,-0.707106781186548,0.707106781186548));
#33004=DIRECTION('ref_axis',(0.,-0.707106781186548,-0.707106781186548));
#33005=DIRECTION('',(0.,0.707106781186547,0.707106781186547));
#33006=DIRECTION('',(-1.,0.,0.));
#33007=DIRECTION('center_axis',(0.,-1.,1.77920356510442E-16));
#33008=DIRECTION('ref_axis',(0.,-1.77920356510442E-16,-1.));
#33009=DIRECTION('',(0.,1.77920356510442E-16,1.));
#33010=DIRECTION('',(-1.,0.,0.));
#33011=DIRECTION('center_axis',(0.,-0.707106781186552,-0.707106781186543));
#33012=DIRECTION('ref_axis',(0.,0.707106781186543,-0.707106781186553));
#33013=DIRECTION('',(0.,-0.707106781186543,0.707106781186552));
#33014=DIRECTION('',(-1.,0.,0.));
#33015=DIRECTION('center_axis',(0.,7.30409884621814E-16,-1.));
#33016=DIRECTION('ref_axis',(0.,1.,7.30409884621814E-16));
#33017=DIRECTION('',(0.,-1.,-7.30409884621814E-16));
#33018=DIRECTION('center_axis',(1.,0.,0.));
#33019=DIRECTION('ref_axis',(0.,0.,-1.));
#33020=DIRECTION('center_axis',(0.,-1.,0.));
#33021=DIRECTION('ref_axis',(0.,0.,-1.));
#33022=DIRECTION('center_axis',(0.,-1.,0.));
#33023=DIRECTION('ref_axis',(0.,0.,-1.));
#33024=DIRECTION('center_axis',(0.,-1.,0.));
#33025=DIRECTION('ref_axis',(0.,0.,-1.));
#33026=DIRECTION('center_axis',(0.,-1.,0.));
#33027=DIRECTION('ref_axis',(0.,0.,-1.));
#33028=DIRECTION('center_axis',(-1.,0.,0.));
#33029=DIRECTION('ref_axis',(0.,0.,1.));
#33030=DIRECTION('',(0.,0.,1.));
#33031=DIRECTION('',(0.,-0.707106781186549,0.707106781186546));
#33032=DIRECTION('',(0.,-1.,0.));
#33033=DIRECTION('',(0.,-0.707106781186547,-0.707106781186548));
#33034=DIRECTION('',(0.,0.,-1.));
#33035=DIRECTION('',(0.,0.707106781186549,-0.707106781186546));
#33036=DIRECTION('',(0.,1.,0.));
#33037=DIRECTION('',(0.,0.707106781186546,0.707106781186549));
#33038=DIRECTION('center_axis',(0.,-1.,0.));
#33039=DIRECTION('ref_axis',(0.,0.,-1.));
#33040=DIRECTION('',(-1.,0.,0.));
#33041=DIRECTION('',(-1.,0.,0.));
#33042=DIRECTION('center_axis',(0.,-0.707106781186546,-0.707106781186549));
#33043=DIRECTION('ref_axis',(0.,0.707106781186549,-0.707106781186546));
#33044=DIRECTION('',(-1.,0.,0.));
#33045=DIRECTION('center_axis',(0.,0.,-1.));
#33046=DIRECTION('ref_axis',(-1.,0.,0.));
#33047=DIRECTION('',(-1.,0.,0.));
#33048=DIRECTION('center_axis',(0.,0.707106781186548,-0.707106781186547));
#33049=DIRECTION('ref_axis',(0.,0.707106781186547,0.707106781186548));
#33050=DIRECTION('',(-1.,0.,0.));
#33051=DIRECTION('center_axis',(0.,1.,0.));
#33052=DIRECTION('ref_axis',(0.,0.,1.));
#33053=DIRECTION('',(-1.,0.,0.));
#33054=DIRECTION('center_axis',(0.,0.707106781186546,0.707106781186549));
#33055=DIRECTION('ref_axis',(0.,-0.707106781186549,0.707106781186546));
#33056=DIRECTION('',(-1.,0.,0.));
#33057=DIRECTION('center_axis',(0.,0.,1.));
#33058=DIRECTION('ref_axis',(1.,0.,0.));
#33059=DIRECTION('',(-1.,0.,0.));
#33060=DIRECTION('center_axis',(0.,-0.707106781186549,0.707106781186546));
#33061=DIRECTION('ref_axis',(0.,-0.707106781186546,-0.707106781186549));
#33062=DIRECTION('center_axis',(1.,0.,0.));
#33063=DIRECTION('ref_axis',(0.,0.,-1.));
#33064=DIRECTION('',(0.,0.500000000000004,-0.866025403784436));
#33065=DIRECTION('',(0.,-0.500000000000004,-0.866025403784436));
#33066=DIRECTION('',(0.,-1.,0.));
#33067=DIRECTION('',(0.,-0.500000000000008,0.866025403784434));
#33068=DIRECTION('',(0.,0.500000000000004,0.866025403784437));
#33069=DIRECTION('',(0.,1.,0.));
#33070=DIRECTION('center_axis',(1.,0.,0.));
#33071=DIRECTION('ref_axis',(0.,0.,-1.));
#33072=DIRECTION('',(0.,0.499999999999999,-0.866025403784439));
#33073=DIRECTION('',(0.,-0.5,-0.866025403784438));
#33074=DIRECTION('',(0.,-1.,0.));
#33075=DIRECTION('',(0.,-0.500000000000001,0.866025403784438));
#33076=DIRECTION('',(0.,0.500000000000001,0.866025403784438));
#33077=DIRECTION('',(0.,1.,0.));
#33078=DIRECTION('center_axis',(1.,0.,0.));
#33079=DIRECTION('ref_axis',(0.,0.,-1.));
#33080=DIRECTION('',(0.,0.5,-0.866025403784439));
#33081=DIRECTION('',(0.,-0.5,-0.866025403784439));
#33082=DIRECTION('',(0.,-1.,0.));
#33083=DIRECTION('',(0.,-0.5,0.866025403784438));
#33084=DIRECTION('',(0.,0.5,0.866025403784438));
#33085=DIRECTION('',(0.,1.,1.00154306582478E-15));
#33086=DIRECTION('center_axis',(1.,0.,0.));
#33087=DIRECTION('ref_axis',(0.,0.,-1.));
#33088=DIRECTION('',(0.,0.500000000000001,-0.866025403784438));
#33089=DIRECTION('',(0.,-0.5,-0.866025403784439));
#33090=DIRECTION('',(0.,-1.,0.));
#33091=DIRECTION('',(0.,-0.5,0.866025403784439));
#33092=DIRECTION('',(0.,0.499999999999999,0.866025403784439));
#33093=DIRECTION('',(0.,1.,-1.00154306582477E-15));
#33094=DIRECTION('center_axis',(0.,-0.866025403784436,-0.500000000000004));
#33095=DIRECTION('ref_axis',(0.,0.500000000000004,-0.866025403784436));
#33096=DIRECTION('',(1.,0.,0.));
#33097=DIRECTION('',(0.,0.500000000000004,-0.866025403784436));
#33098=DIRECTION('',(1.,0.,0.));
#33099=DIRECTION('center_axis',(0.,-0.866025403784436,0.500000000000004));
#33100=DIRECTION('ref_axis',(0.,-0.500000000000004,-0.866025403784436));
#33101=DIRECTION('',(0.,-0.500000000000004,-0.866025403784436));
#33102=DIRECTION('',(1.,0.,0.));
#33103=DIRECTION('center_axis',(0.,0.,1.));
#33104=DIRECTION('ref_axis',(1.,0.,0.));
#33105=DIRECTION('',(0.,-1.,0.));
#33106=DIRECTION('',(1.,0.,0.));
#33107=DIRECTION('center_axis',(0.,0.866025403784434,0.500000000000008));
#33108=DIRECTION('ref_axis',(0.,-0.500000000000007,0.866025403784434));
#33109=DIRECTION('',(0.,-0.500000000000008,0.866025403784434));
#33110=DIRECTION('',(1.,0.,0.));
#33111=DIRECTION('center_axis',(0.,0.866025403784437,-0.500000000000004));
#33112=DIRECTION('ref_axis',(0.,0.500000000000004,0.866025403784437));
#33113=DIRECTION('',(0.,0.500000000000004,0.866025403784437));
#33114=DIRECTION('',(1.,0.,0.));
#33115=DIRECTION('center_axis',(0.,0.,-1.));
#33116=DIRECTION('ref_axis',(-1.,0.,0.));
#33117=DIRECTION('',(0.,1.,0.));
#33118=DIRECTION('center_axis',(1.,0.,0.));
#33119=DIRECTION('ref_axis',(0.,0.,-1.));
#33120=DIRECTION('center_axis',(0.,-0.866025403784439,-0.499999999999999));
#33121=DIRECTION('ref_axis',(0.,0.499999999999999,-0.866025403784439));
#33122=DIRECTION('',(1.,0.,0.));
#33123=DIRECTION('',(0.,0.499999999999999,-0.866025403784439));
#33124=DIRECTION('',(1.,0.,0.));
#33125=DIRECTION('center_axis',(0.,-0.866025403784438,0.5));
#33126=DIRECTION('ref_axis',(0.,-0.5,-0.866025403784438));
#33127=DIRECTION('',(0.,-0.5,-0.866025403784438));
#33128=DIRECTION('',(1.,0.,0.));
#33129=DIRECTION('center_axis',(0.,0.,1.));
#33130=DIRECTION('ref_axis',(1.,0.,0.));
#33131=DIRECTION('',(0.,-1.,0.));
#33132=DIRECTION('',(1.,0.,0.));
#33133=DIRECTION('center_axis',(0.,0.866025403784438,0.500000000000001));
#33134=DIRECTION('ref_axis',(0.,-0.500000000000001,0.866025403784438));
#33135=DIRECTION('',(0.,-0.500000000000001,0.866025403784438));
#33136=DIRECTION('',(1.,0.,0.));
#33137=DIRECTION('center_axis',(0.,0.866025403784438,-0.500000000000001));
#33138=DIRECTION('ref_axis',(0.,0.500000000000001,0.866025403784438));
#33139=DIRECTION('',(0.,0.500000000000001,0.866025403784438));
#33140=DIRECTION('',(1.,0.,0.));
#33141=DIRECTION('center_axis',(0.,0.,-1.));
#33142=DIRECTION('ref_axis',(-1.,0.,0.));
#33143=DIRECTION('',(0.,1.,0.));
#33144=DIRECTION('center_axis',(1.,0.,0.));
#33145=DIRECTION('ref_axis',(0.,0.,-1.));
#33146=DIRECTION('center_axis',(0.,-0.866025403784438,-0.500000000000001));
#33147=DIRECTION('ref_axis',(0.,0.500000000000001,-0.866025403784438));
#33148=DIRECTION('',(1.,0.,0.));
#33149=DIRECTION('',(0.,0.500000000000001,-0.866025403784438));
#33150=DIRECTION('',(1.,0.,0.));
#33151=DIRECTION('center_axis',(0.,-0.866025403784439,0.5));
#33152=DIRECTION('ref_axis',(0.,-0.5,-0.866025403784439));
#33153=DIRECTION('',(0.,-0.5,-0.866025403784439));
#33154=DIRECTION('',(1.,0.,0.));
#33155=DIRECTION('center_axis',(0.,0.,1.));
#33156=DIRECTION('ref_axis',(1.,0.,0.));
#33157=DIRECTION('',(0.,-1.,0.));
#33158=DIRECTION('',(1.,0.,0.));
#33159=DIRECTION('center_axis',(0.,0.866025403784439,0.5));
#33160=DIRECTION('ref_axis',(0.,-0.5,0.866025403784439));
#33161=DIRECTION('',(0.,-0.5,0.866025403784439));
#33162=DIRECTION('',(1.,0.,0.));
#33163=DIRECTION('center_axis',(0.,0.866025403784439,-0.499999999999999));
#33164=DIRECTION('ref_axis',(0.,0.499999999999999,0.866025403784439));
#33165=DIRECTION('',(0.,0.499999999999999,0.866025403784439));
#33166=DIRECTION('',(1.,0.,0.));
#33167=DIRECTION('center_axis',(0.,-1.00154306582477E-15,-1.));
#33168=DIRECTION('ref_axis',(0.,1.,-1.00154306582477E-15));
#33169=DIRECTION('',(0.,1.,-1.00154306582477E-15));
#33170=DIRECTION('center_axis',(1.,0.,0.));
#33171=DIRECTION('ref_axis',(0.,0.,-1.));
#33172=DIRECTION('center_axis',(0.,-0.866025403784439,-0.5));
#33173=DIRECTION('ref_axis',(0.,0.5,-0.866025403784439));
#33174=DIRECTION('',(1.,0.,0.));
#33175=DIRECTION('',(0.,0.5,-0.866025403784439));
#33176=DIRECTION('',(1.,0.,0.));
#33177=DIRECTION('center_axis',(0.,-0.866025403784439,0.5));
#33178=DIRECTION('ref_axis',(0.,-0.5,-0.866025403784439));
#33179=DIRECTION('',(0.,-0.5,-0.866025403784439));
#33180=DIRECTION('',(1.,0.,0.));
#33181=DIRECTION('center_axis',(0.,0.,1.));
#33182=DIRECTION('ref_axis',(1.,0.,0.));
#33183=DIRECTION('',(0.,-1.,0.));
#33184=DIRECTION('',(1.,0.,0.));
#33185=DIRECTION('center_axis',(0.,0.866025403784438,0.5));
#33186=DIRECTION('ref_axis',(0.,-0.5,0.866025403784438));
#33187=DIRECTION('',(0.,-0.5,0.866025403784438));
#33188=DIRECTION('',(1.,0.,0.));
#33189=DIRECTION('center_axis',(0.,0.866025403784438,-0.5));
#33190=DIRECTION('ref_axis',(0.,0.5,0.866025403784438));
#33191=DIRECTION('',(0.,0.5,0.866025403784438));
#33192=DIRECTION('',(1.,0.,0.));
#33193=DIRECTION('center_axis',(0.,1.00154306582478E-15,-1.));
#33194=DIRECTION('ref_axis',(0.,1.,1.00154306582478E-15));
#33195=DIRECTION('',(0.,1.,1.00154306582478E-15));
#33196=DIRECTION('center_axis',(1.,0.,0.));
#33197=DIRECTION('ref_axis',(0.,0.,-1.));
#33198=DIRECTION('center_axis',(1.,0.,0.));
#33199=DIRECTION('ref_axis',(0.,0.,-1.));
#33200=DIRECTION('center_axis',(1.,0.,0.));
#33201=DIRECTION('ref_axis',(0.,0.,-1.));
#33202=DIRECTION('center_axis',(-1.,0.,0.));
#33203=DIRECTION('ref_axis',(0.,0.,1.));
#33204=DIRECTION('center_axis',(-1.,0.,0.));
#33205=DIRECTION('ref_axis',(0.,0.,1.));
#40424=CARTESIAN_POINT('',(0.,0.,0.));
#40425=CARTESIAN_POINT('Origin',(33.,28.,0.));
#40426=CARTESIAN_POINT('',(27.,28.,14.));
#40427=CARTESIAN_POINT('Origin',(27.,28.,0.));
#40428=CARTESIAN_POINT('',(33.,28.,14.));
#40429=CARTESIAN_POINT('',(33.,28.,14.));
#40430=CARTESIAN_POINT('Origin',(33.,28.,0.));
#40431=CARTESIAN_POINT('Origin',(33.,28.,0.));
#40432=CARTESIAN_POINT('',(24.,28.,9.75));
#40433=CARTESIAN_POINT('Origin',(24.,28.,0.));
#40434=CARTESIAN_POINT('',(27.,28.,9.75));
#40435=CARTESIAN_POINT('',(33.,28.,9.75));
#40436=CARTESIAN_POINT('Origin',(27.,28.,0.));
#40437=CARTESIAN_POINT('Origin',(33.,28.,0.));
#40438=CARTESIAN_POINT('',(6.,28.,7.5));
#40439=CARTESIAN_POINT('Origin',(6.,28.,0.));
#40440=CARTESIAN_POINT('',(24.,28.,7.5));
#40441=CARTESIAN_POINT('',(33.,28.,7.5));
#40442=CARTESIAN_POINT('Origin',(24.,28.,0.));
#40443=CARTESIAN_POINT('Origin',(33.,28.,0.));
#40444=CARTESIAN_POINT('',(2.,28.,9.75));
#40445=CARTESIAN_POINT('Origin',(2.,28.,0.));
#40446=CARTESIAN_POINT('',(6.,28.,9.75));
#40447=CARTESIAN_POINT('',(33.,28.,9.75));
#40448=CARTESIAN_POINT('Origin',(6.,28.,0.));
#40449=CARTESIAN_POINT('Origin',(33.,28.,0.));
#40450=CARTESIAN_POINT('',(0.,28.,14.));
#40451=CARTESIAN_POINT('Origin',(0.,28.,0.));
#40452=CARTESIAN_POINT('',(2.,28.,14.));
#40453=CARTESIAN_POINT('',(33.,28.,14.));
#40454=CARTESIAN_POINT('Origin',(2.,28.,0.));
#40455=CARTESIAN_POINT('Origin',(33.,14.2114177668623,13.7885822331377));
#40456=CARTESIAN_POINT('',(27.,14.2114177668623,10.6885822331377));
#40457=CARTESIAN_POINT('Origin',(27.,14.2114177668623,13.7885822331377));
#40458=CARTESIAN_POINT('',(33.,14.2114177668623,10.6885822331377));
#40459=CARTESIAN_POINT('',(33.,14.2114177668623,10.6885822331377));
#40460=CARTESIAN_POINT('Origin',(33.,14.2114177668623,13.7885822331377));
#40461=CARTESIAN_POINT('Origin',(33.,14.2114177668623,-13.7885822331377));
#40462=CARTESIAN_POINT('',(27.,14.2114177668623,-16.8885822331377));
#40463=CARTESIAN_POINT('Origin',(27.,14.2114177668623,-13.7885822331377));
#40464=CARTESIAN_POINT('',(33.,14.2114177668623,-16.8885822331377));
#40465=CARTESIAN_POINT('',(33.,14.2114177668623,-16.8885822331377));
#40466=CARTESIAN_POINT('Origin',(33.,14.2114177668623,-13.7885822331377));
#40467=CARTESIAN_POINT('Origin',(33.,41.7885822331377,-13.7885822331377));
#40468=CARTESIAN_POINT('',(27.,41.7885822331377,-16.8885822331377));
#40469=CARTESIAN_POINT('Origin',(27.,41.7885822331377,-13.7885822331377));
#40470=CARTESIAN_POINT('',(33.,41.7885822331377,-16.8885822331377));
#40471=CARTESIAN_POINT('',(33.,41.7885822331377,-16.8885822331377));
#40472=CARTESIAN_POINT('Origin',(33.,41.7885822331377,-13.7885822331377));
#40473=CARTESIAN_POINT('Origin',(33.,41.7885822331377,13.7885822331377));
#40474=CARTESIAN_POINT('',(27.,41.7885822331377,10.6885822331377));
#40475=CARTESIAN_POINT('Origin',(27.,41.7885822331377,13.7885822331377));
#40476=CARTESIAN_POINT('',(33.,41.7885822331377,10.6885822331377));
#40477=CARTESIAN_POINT('',(33.,41.7885822331377,10.6885822331377));
#40478=CARTESIAN_POINT('Origin',(33.,41.7885822331377,13.7885822331377));
#40479=CARTESIAN_POINT('Origin',(33.,14.2114177668623,-13.7885822331377));
#40480=CARTESIAN_POINT('',(33.,14.2114177668623,-17.2885822331377));
#40481=CARTESIAN_POINT('Origin',(33.,14.2114177668623,-13.7885822331377));
#40482=CARTESIAN_POINT('',(27.,14.2114177668623,-17.2885822331377));
#40483=CARTESIAN_POINT('',(33.,14.2114177668623,-17.2885822331377));
#40484=CARTESIAN_POINT('Origin',(27.,14.2114177668623,-13.7885822331377));
#40485=CARTESIAN_POINT('Origin',(33.,14.2114177668623,13.7885822331377));
#40486=CARTESIAN_POINT('',(33.,14.2114177668623,10.2885822331377));
#40487=CARTESIAN_POINT('Origin',(33.,14.2114177668623,13.7885822331377));
#40488=CARTESIAN_POINT('',(27.,14.2114177668623,10.2885822331377));
#40489=CARTESIAN_POINT('',(33.,14.2114177668623,10.2885822331377));
#40490=CARTESIAN_POINT('Origin',(27.,14.2114177668623,13.7885822331377));
#40491=CARTESIAN_POINT('Origin',(33.,41.7885822331377,-13.7885822331377));
#40492=CARTESIAN_POINT('',(33.,41.7885822331377,-17.2885822331377));
#40493=CARTESIAN_POINT('Origin',(33.,41.7885822331377,-13.7885822331377));
#40494=CARTESIAN_POINT('',(27.,41.7885822331377,-17.2885822331377));
#40495=CARTESIAN_POINT('',(33.,41.7885822331377,-17.2885822331377));
#40496=CARTESIAN_POINT('Origin',(27.,41.7885822331377,-13.7885822331377));
#40497=CARTESIAN_POINT('Origin',(33.,41.7885822331377,13.7885822331377));
#40498=CARTESIAN_POINT('',(33.,41.7885822331377,10.2885822331377));
#40499=CARTESIAN_POINT('Origin',(33.,41.7885822331377,13.7885822331377));
#40500=CARTESIAN_POINT('',(27.,41.7885822331377,10.2885822331377));
#40501=CARTESIAN_POINT('',(33.,41.7885822331377,10.2885822331377));
#40502=CARTESIAN_POINT('Origin',(27.,41.7885822331377,13.7885822331377));
#40503=CARTESIAN_POINT('Origin',(6.,38.,-27.));
#40504=CARTESIAN_POINT('',(5.99999999999999,31.5,-32.5));
#40505=CARTESIAN_POINT('Origin',(6.,31.5,-27.));
#40506=CARTESIAN_POINT('',(5.99999999999999,38.,-32.5));
#40507=CARTESIAN_POINT('',(5.99999999999999,38.,-32.5));
#40508=CARTESIAN_POINT('Origin',(6.,38.,-27.));
#40509=CARTESIAN_POINT('Origin',(6.,38.,-27.));
#40510=CARTESIAN_POINT('',(6.,0.,-30.3));
#40511=CARTESIAN_POINT('Origin',(6.,0.,-27.));
#40512=CARTESIAN_POINT('',(6.,31.5,-30.3));
#40513=CARTESIAN_POINT('',(6.,38.,-30.3));
#40514=CARTESIAN_POINT('Origin',(6.,31.5,-27.));
#40515=CARTESIAN_POINT('Origin',(6.,38.,27.));
#40516=CARTESIAN_POINT('',(5.99999999999999,31.5,21.5));
#40517=CARTESIAN_POINT('Origin',(6.,31.5,27.));
#40518=CARTESIAN_POINT('',(5.99999999999999,38.,21.5));
#40519=CARTESIAN_POINT('',(5.99999999999999,38.,21.5));
#40520=CARTESIAN_POINT('Origin',(6.,38.,27.));
#40521=CARTESIAN_POINT('Origin',(6.,38.,27.));
#40522=CARTESIAN_POINT('',(6.,0.,23.7));
#40523=CARTESIAN_POINT('Origin',(6.,0.,27.));
#40524=CARTESIAN_POINT('',(6.,31.5,23.7));
#40525=CARTESIAN_POINT('',(6.,38.,23.7));
#40526=CARTESIAN_POINT('Origin',(6.,31.5,27.));
#40527=CARTESIAN_POINT('Origin',(21.,38.,-27.));
#40528=CARTESIAN_POINT('',(21.,31.5,-32.5));
#40529=CARTESIAN_POINT('Origin',(21.,31.5,-27.));
#40530=CARTESIAN_POINT('',(21.,38.,-32.5));
#40531=CARTESIAN_POINT('',(21.,38.,-32.5));
#40532=CARTESIAN_POINT('Origin',(21.,38.,-27.));
#40533=CARTESIAN_POINT('Origin',(21.,38.,-27.));
#40534=CARTESIAN_POINT('',(21.,0.,-30.3));
#40535=CARTESIAN_POINT('Origin',(21.,0.,-27.));
#40536=CARTESIAN_POINT('',(21.,31.5,-30.3));
#40537=CARTESIAN_POINT('',(21.,38.,-30.3));
#40538=CARTESIAN_POINT('Origin',(21.,31.5,-27.));
#40539=CARTESIAN_POINT('Origin',(21.,38.,27.));
#40540=CARTESIAN_POINT('',(21.,31.5,21.5));
#40541=CARTESIAN_POINT('Origin',(21.,31.5,27.));
#40542=CARTESIAN_POINT('',(21.,38.,21.5));
#40543=CARTESIAN_POINT('',(21.,38.,21.5));
#40544=CARTESIAN_POINT('Origin',(21.,38.,27.));
#40545=CARTESIAN_POINT('Origin',(21.,38.,27.));
#40546=CARTESIAN_POINT('',(21.,0.,23.7));
#40547=CARTESIAN_POINT('Origin',(21.,0.,27.));
#40548=CARTESIAN_POINT('',(21.,31.5,23.7));
#40549=CARTESIAN_POINT('',(21.,38.,23.7));
#40550=CARTESIAN_POINT('Origin',(21.,31.5,27.));
#40551=CARTESIAN_POINT('Origin',(27.,0.,0.));
#40552=CARTESIAN_POINT('Origin',(27.,0.,0.));
#40553=CARTESIAN_POINT('Origin',(27.,0.,0.));
#40554=CARTESIAN_POINT('Origin',(27.,0.,0.));
#40555=CARTESIAN_POINT('Origin',(27.,0.,0.));
#40556=CARTESIAN_POINT('',(27.,38.,20.));
#40557=CARTESIAN_POINT('',(27.,38.,34.5));
#40558=CARTESIAN_POINT('',(27.,38.,20.));
#40559=CARTESIAN_POINT('',(27.,37.5,35.));
#40560=CARTESIAN_POINT('',(27.,38.,34.5));
#40561=CARTESIAN_POINT('',(27.,0.,35.));
#40562=CARTESIAN_POINT('',(27.,37.5,35.));
#40563=CARTESIAN_POINT('',(27.,1.53660089149199E-14,-35.));
#40564=CARTESIAN_POINT('',(27.,0.,35.));
#40565=CARTESIAN_POINT('',(27.,37.5,-35.));
#40566=CARTESIAN_POINT('',(27.,37.5,-35.));
#40567=CARTESIAN_POINT('',(27.,38.,-34.5));
#40568=CARTESIAN_POINT('',(27.,38.,-34.5));
#40569=CARTESIAN_POINT('',(27.,38.,-20.));
#40570=CARTESIAN_POINT('',(27.,38.,-20.));
#40571=CARTESIAN_POINT('',(27.,47.5,-20.));
#40572=CARTESIAN_POINT('',(27.,47.5,-20.));
#40573=CARTESIAN_POINT('',(27.,48.,-19.5));
#40574=CARTESIAN_POINT('',(27.,48.,-19.5));
#40575=CARTESIAN_POINT('',(27.,48.,19.5));
#40576=CARTESIAN_POINT('',(27.,48.,19.5));
#40577=CARTESIAN_POINT('',(27.,47.5,20.));
#40578=CARTESIAN_POINT('',(27.,47.5,20.));
#40579=CARTESIAN_POINT('',(27.,47.5,20.));
#40580=CARTESIAN_POINT('',(27.,47.,17.));
#40581=CARTESIAN_POINT('',(27.,45.,19.));
#40582=CARTESIAN_POINT('',(27.,45.,19.));
#40583=CARTESIAN_POINT('',(27.,47.,-17.));
#40584=CARTESIAN_POINT('',(27.,47.,17.));
#40585=CARTESIAN_POINT('',(27.,45.,-19.));
#40586=CARTESIAN_POINT('',(27.,47.,-17.));
#40587=CARTESIAN_POINT('',(27.,11.,-19.));
#40588=CARTESIAN_POINT('',(27.,45.,-19.));
#40589=CARTESIAN_POINT('',(27.,9.,-17.));
#40590=CARTESIAN_POINT('',(27.,11.,-19.));
#40591=CARTESIAN_POINT('',(27.,9.,17.));
#40592=CARTESIAN_POINT('',(27.,9.,17.));
#40593=CARTESIAN_POINT('',(27.,11.,19.));
#40594=CARTESIAN_POINT('',(27.,11.,19.));
#40595=CARTESIAN_POINT('',(27.,45.,19.));
#40596=CARTESIAN_POINT('Origin',(27.,38.,20.));
#40597=CARTESIAN_POINT('',(0.,38.,20.));
#40598=CARTESIAN_POINT('',(0.,38.,34.5));
#40599=CARTESIAN_POINT('',(0.,38.,20.));
#40600=CARTESIAN_POINT('',(27.,38.,34.5));
#40601=CARTESIAN_POINT('',(27.,38.,20.));
#40602=CARTESIAN_POINT('Origin',(27.,38.,34.5));
#40603=CARTESIAN_POINT('',(0.,37.5,35.));
#40604=CARTESIAN_POINT('',(0.,38.,34.5));
#40605=CARTESIAN_POINT('',(27.,37.5,35.));
#40606=CARTESIAN_POINT('Origin',(27.,37.5,35.));
#40607=CARTESIAN_POINT('',(0.,0.,35.));
#40608=CARTESIAN_POINT('',(0.,37.5,35.));
#40609=CARTESIAN_POINT('',(27.,0.,35.));
#40610=CARTESIAN_POINT('Origin',(27.,0.,35.));
#40611=CARTESIAN_POINT('',(0.,1.53660089149199E-14,-35.));
#40612=CARTESIAN_POINT('',(0.,0.,35.));
#40613=CARTESIAN_POINT('',(27.,1.53660089149199E-14,-35.));
#40614=CARTESIAN_POINT('Origin',(27.,37.5,-35.));
#40615=CARTESIAN_POINT('',(0.,37.5,-35.));
#40616=CARTESIAN_POINT('',(0.,37.5,-35.));
#40617=CARTESIAN_POINT('',(27.,37.5,-35.));
#40618=CARTESIAN_POINT('Origin',(27.,38.,-34.5));
#40619=CARTESIAN_POINT('',(0.,38.,-34.5));
#40620=CARTESIAN_POINT('',(0.,38.,-34.5));
#40621=CARTESIAN_POINT('',(27.,38.,-34.5));
#40622=CARTESIAN_POINT('Origin',(27.,38.,-20.));
#40623=CARTESIAN_POINT('',(0.,38.,-20.));
#40624=CARTESIAN_POINT('',(0.,38.,-20.));
#40625=CARTESIAN_POINT('',(27.,38.,-20.));
#40626=CARTESIAN_POINT('Origin',(27.,47.5,-20.));
#40627=CARTESIAN_POINT('',(0.,47.5,-20.));
#40628=CARTESIAN_POINT('',(0.,47.5,-20.));
#40629=CARTESIAN_POINT('',(27.,47.5,-20.));
#40630=CARTESIAN_POINT('Origin',(27.,48.,-19.5));
#40631=CARTESIAN_POINT('',(0.,48.,-19.5));
#40632=CARTESIAN_POINT('',(0.,48.,-19.5));
#40633=CARTESIAN_POINT('',(27.,48.,-19.5));
#40634=CARTESIAN_POINT('Origin',(27.,48.,19.5));
#40635=CARTESIAN_POINT('',(0.,48.,19.5));
#40636=CARTESIAN_POINT('',(0.,48.,19.5));
#40637=CARTESIAN_POINT('',(27.,48.,19.5));
#40638=CARTESIAN_POINT('Origin',(27.,47.5,20.));
#40639=CARTESIAN_POINT('',(0.,47.5,20.));
#40640=CARTESIAN_POINT('',(0.,47.5,20.));
#40641=CARTESIAN_POINT('',(27.,47.5,20.));
#40642=CARTESIAN_POINT('Origin',(27.,47.5,20.));
#40643=CARTESIAN_POINT('',(0.,47.5,20.));
#40644=CARTESIAN_POINT('Origin',(0.,0.,0.));
#40645=CARTESIAN_POINT('Origin',(24.3,31.5,27.));
#40646=CARTESIAN_POINT('Origin',(24.3,31.5,-27.));
#40647=CARTESIAN_POINT('Origin',(9.3,31.5,27.));
#40648=CARTESIAN_POINT('Origin',(9.3,31.5,-27.));
#40649=CARTESIAN_POINT('Origin',(33.,0.,0.));
#40650=CARTESIAN_POINT('',(33.,47.,-17.));
#40651=CARTESIAN_POINT('',(33.,47.,17.));
#40652=CARTESIAN_POINT('',(33.,47.,17.));
#40653=CARTESIAN_POINT('',(33.,45.,19.));
#40654=CARTESIAN_POINT('',(33.,45.,19.));
#40655=CARTESIAN_POINT('',(33.,11.,19.));
#40656=CARTESIAN_POINT('',(33.,45.,19.));
#40657=CARTESIAN_POINT('',(33.,9.,17.));
#40658=CARTESIAN_POINT('',(33.,11.,19.));
#40659=CARTESIAN_POINT('',(33.,9.,-17.));
#40660=CARTESIAN_POINT('',(33.,9.,17.));
#40661=CARTESIAN_POINT('',(33.,11.,-19.));
#40662=CARTESIAN_POINT('',(33.,11.,-19.));
#40663=CARTESIAN_POINT('',(33.,45.,-19.));
#40664=CARTESIAN_POINT('',(33.,45.,-19.));
#40665=CARTESIAN_POINT('',(33.,47.,-17.));
#40666=CARTESIAN_POINT('Origin',(33.,47.,17.));
#40667=CARTESIAN_POINT('',(33.,47.,17.));
#40668=CARTESIAN_POINT('',(33.,47.,-17.));
#40669=CARTESIAN_POINT('Origin',(33.,45.,19.));
#40670=CARTESIAN_POINT('',(33.,45.,19.));
#40671=CARTESIAN_POINT('Origin',(33.,45.,19.));
#40672=CARTESIAN_POINT('',(33.,11.,19.));
#40673=CARTESIAN_POINT('Origin',(33.,11.,19.));
#40674=CARTESIAN_POINT('',(33.,9.,17.));
#40675=CARTESIAN_POINT('Origin',(33.,9.,17.));
#40676=CARTESIAN_POINT('',(33.,9.,-17.));
#40677=CARTESIAN_POINT('Origin',(33.,11.,-19.));
#40678=CARTESIAN_POINT('',(33.,11.,-19.));
#40679=CARTESIAN_POINT('Origin',(33.,45.,-19.));
#40680=CARTESIAN_POINT('',(33.,45.,-19.));
#40681=CARTESIAN_POINT('Origin',(33.,47.,-17.));
#40682=CARTESIAN_POINT('Origin',(33.,41.7885822331377,13.7885822331377));
#40683=CARTESIAN_POINT('',(33.,40.0565314255688,13.7885822331377));
#40684=CARTESIAN_POINT('',(33.,40.9225568293532,12.2885822331377));
#40685=CARTESIAN_POINT('',(33.,40.0565314255688,13.7885822331377));
#40686=CARTESIAN_POINT('',(33.,40.9225568293533,15.2885822331377));
#40687=CARTESIAN_POINT('',(33.,40.9225568293533,15.2885822331377));
#40688=CARTESIAN_POINT('',(33.,42.6546076369221,15.2885822331377));
#40689=CARTESIAN_POINT('',(33.,42.6546076369221,15.2885822331377));
#40690=CARTESIAN_POINT('',(33.,43.5206330407066,13.7885822331377));
#40691=CARTESIAN_POINT('',(33.,43.5206330407066,13.7885822331377));
#40692=CARTESIAN_POINT('',(33.,42.6546076369221,12.2885822331377));
#40693=CARTESIAN_POINT('',(33.,42.6546076369221,12.2885822331377));
#40694=CARTESIAN_POINT('',(33.,40.9225568293532,12.2885822331377));
#40695=CARTESIAN_POINT('Origin',(33.,41.7885822331377,-13.7885822331377));
#40696=CARTESIAN_POINT('',(33.,40.0565314255688,-13.7885822331377));
#40697=CARTESIAN_POINT('',(33.,40.9225568293532,-15.2885822331377));
#40698=CARTESIAN_POINT('',(33.,40.0565314255688,-13.7885822331377));
#40699=CARTESIAN_POINT('',(33.,40.9225568293532,-12.2885822331377));
#40700=CARTESIAN_POINT('',(33.,40.9225568293532,-12.2885822331377));
#40701=CARTESIAN_POINT('',(33.,42.6546076369221,-12.2885822331377));
#40702=CARTESIAN_POINT('',(33.,42.6546076369221,-12.2885822331377));
#40703=CARTESIAN_POINT('',(33.,43.5206330407065,-13.7885822331377));
#40704=CARTESIAN_POINT('',(33.,43.5206330407065,-13.7885822331377));
#40705=CARTESIAN_POINT('',(33.,42.6546076369221,-15.2885822331377));
#40706=CARTESIAN_POINT('',(33.,42.6546076369221,-15.2885822331377));
#40707=CARTESIAN_POINT('',(33.,40.9225568293532,-15.2885822331377));
#40708=CARTESIAN_POINT('Origin',(33.,14.2114177668623,-13.7885822331377));
#40709=CARTESIAN_POINT('',(33.,12.4793669592934,-13.7885822331377));
#40710=CARTESIAN_POINT('',(33.,13.3453923630779,-15.2885822331377));
#40711=CARTESIAN_POINT('',(33.,12.4793669592934,-13.7885822331377));
#40712=CARTESIAN_POINT('',(33.,13.3453923630779,-12.2885822331377));
#40713=CARTESIAN_POINT('',(33.,13.3453923630779,-12.2885822331377));
#40714=CARTESIAN_POINT('',(33.,15.0774431706468,-12.2885822331377));
#40715=CARTESIAN_POINT('',(33.,15.0774431706468,-12.2885822331377));
#40716=CARTESIAN_POINT('',(33.,15.9434685744312,-13.7885822331377));
#40717=CARTESIAN_POINT('',(33.,15.9434685744312,-13.7885822331377));
#40718=CARTESIAN_POINT('',(33.,15.0774431706468,-15.2885822331377));
#40719=CARTESIAN_POINT('',(33.,15.0774431706468,-15.2885822331377));
#40720=CARTESIAN_POINT('',(33.,13.3453923630779,-15.2885822331377));
#40721=CARTESIAN_POINT('Origin',(33.,14.2114177668623,13.7885822331377));
#40722=CARTESIAN_POINT('',(33.,12.4793669592934,13.7885822331377));
#40723=CARTESIAN_POINT('',(33.,13.3453923630779,12.2885822331377));
#40724=CARTESIAN_POINT('',(33.,12.4793669592934,13.7885822331377));
#40725=CARTESIAN_POINT('',(33.,13.3453923630779,15.2885822331377));
#40726=CARTESIAN_POINT('',(33.,13.3453923630779,15.2885822331377));
#40727=CARTESIAN_POINT('',(33.,15.0774431706468,15.2885822331377));
#40728=CARTESIAN_POINT('',(33.,15.0774431706468,15.2885822331377));
#40729=CARTESIAN_POINT('',(33.,15.9434685744312,13.7885822331377));
#40730=CARTESIAN_POINT('',(33.,15.9434685744312,13.7885822331377));
#40731=CARTESIAN_POINT('',(33.,15.0774431706468,12.2885822331377));
#40732=CARTESIAN_POINT('',(33.,15.0774431706468,12.2885822331377));
#40733=CARTESIAN_POINT('',(33.,13.3453923630779,12.2885822331377));
#40734=CARTESIAN_POINT('Origin',(30.,40.0565314255688,13.7885822331377));
#40735=CARTESIAN_POINT('',(30.,40.9225568293532,12.2885822331377));
#40736=CARTESIAN_POINT('',(30.,40.9225568293532,12.2885822331377));
#40737=CARTESIAN_POINT('',(30.,40.0565314255688,13.7885822331377));
#40738=CARTESIAN_POINT('',(30.,40.0565314255688,13.7885822331377));
#40739=CARTESIAN_POINT('',(30.,40.0565314255688,13.7885822331377));
#40740=CARTESIAN_POINT('Origin',(30.,40.9225568293533,15.2885822331377));
#40741=CARTESIAN_POINT('',(30.,40.9225568293533,15.2885822331377));
#40742=CARTESIAN_POINT('',(30.,40.9225568293533,15.2885822331377));
#40743=CARTESIAN_POINT('',(30.,40.9225568293533,15.2885822331377));
#40744=CARTESIAN_POINT('Origin',(30.,42.6546076369221,15.2885822331377));
#40745=CARTESIAN_POINT('',(30.,42.6546076369221,15.2885822331377));
#40746=CARTESIAN_POINT('',(30.,42.6546076369221,15.2885822331377));
#40747=CARTESIAN_POINT('',(30.,42.6546076369221,15.2885822331377));
#40748=CARTESIAN_POINT('Origin',(30.,43.5206330407066,13.7885822331377));
#40749=CARTESIAN_POINT('',(30.,43.5206330407066,13.7885822331377));
#40750=CARTESIAN_POINT('',(30.,43.5206330407066,13.7885822331377));
#40751=CARTESIAN_POINT('',(30.,43.5206330407066,13.7885822331377));
#40752=CARTESIAN_POINT('Origin',(30.,42.6546076369221,12.2885822331377));
#40753=CARTESIAN_POINT('',(30.,42.6546076369221,12.2885822331377));
#40754=CARTESIAN_POINT('',(30.,42.6546076369221,12.2885822331377));
#40755=CARTESIAN_POINT('',(30.,42.6546076369221,12.2885822331377));
#40756=CARTESIAN_POINT('Origin',(30.,40.9225568293532,12.2885822331377));
#40757=CARTESIAN_POINT('',(30.,40.9225568293532,12.2885822331377));
#40758=CARTESIAN_POINT('Origin',(30.,0.,0.));
#40759=CARTESIAN_POINT('Origin',(30.,40.0565314255688,-13.7885822331377));
#40760=CARTESIAN_POINT('',(30.,40.9225568293532,-15.2885822331377));
#40761=CARTESIAN_POINT('',(30.,40.9225568293532,-15.2885822331377));
#40762=CARTESIAN_POINT('',(30.,40.0565314255688,-13.7885822331377));
#40763=CARTESIAN_POINT('',(30.,40.0565314255688,-13.7885822331377));
#40764=CARTESIAN_POINT('',(30.,40.0565314255688,-13.7885822331377));
#40765=CARTESIAN_POINT('Origin',(30.,40.9225568293532,-12.2885822331377));
#40766=CARTESIAN_POINT('',(30.,40.9225568293532,-12.2885822331377));
#40767=CARTESIAN_POINT('',(30.,40.9225568293532,-12.2885822331377));
#40768=CARTESIAN_POINT('',(30.,40.9225568293532,-12.2885822331377));
#40769=CARTESIAN_POINT('Origin',(30.,42.6546076369221,-12.2885822331377));
#40770=CARTESIAN_POINT('',(30.,42.6546076369221,-12.2885822331377));
#40771=CARTESIAN_POINT('',(30.,42.6546076369221,-12.2885822331377));
#40772=CARTESIAN_POINT('',(30.,42.6546076369221,-12.2885822331377));
#40773=CARTESIAN_POINT('Origin',(30.,43.5206330407065,-13.7885822331377));
#40774=CARTESIAN_POINT('',(30.,43.5206330407065,-13.7885822331377));
#40775=CARTESIAN_POINT('',(30.,43.5206330407065,-13.7885822331377));
#40776=CARTESIAN_POINT('',(30.,43.5206330407065,-13.7885822331377));
#40777=CARTESIAN_POINT('Origin',(30.,42.6546076369221,-15.2885822331377));
#40778=CARTESIAN_POINT('',(30.,42.6546076369221,-15.2885822331377));
#40779=CARTESIAN_POINT('',(30.,42.6546076369221,-15.2885822331377));
#40780=CARTESIAN_POINT('',(30.,42.6546076369221,-15.2885822331377));
#40781=CARTESIAN_POINT('Origin',(30.,40.9225568293532,-15.2885822331377));
#40782=CARTESIAN_POINT('',(30.,40.9225568293532,-15.2885822331377));
#40783=CARTESIAN_POINT('Origin',(30.,0.,0.));
#40784=CARTESIAN_POINT('Origin',(30.,12.4793669592934,13.7885822331377));
#40785=CARTESIAN_POINT('',(30.,13.3453923630779,12.2885822331377));
#40786=CARTESIAN_POINT('',(30.,13.3453923630779,12.2885822331377));
#40787=CARTESIAN_POINT('',(30.,12.4793669592934,13.7885822331377));
#40788=CARTESIAN_POINT('',(30.,12.4793669592934,13.7885822331377));
#40789=CARTESIAN_POINT('',(30.,12.4793669592934,13.7885822331377));
#40790=CARTESIAN_POINT('Origin',(30.,13.3453923630779,15.2885822331377));
#40791=CARTESIAN_POINT('',(30.,13.3453923630779,15.2885822331377));
#40792=CARTESIAN_POINT('',(30.,13.3453923630779,15.2885822331377));
#40793=CARTESIAN_POINT('',(30.,13.3453923630779,15.2885822331377));
#40794=CARTESIAN_POINT('Origin',(30.,15.0774431706468,15.2885822331377));
#40795=CARTESIAN_POINT('',(30.,15.0774431706468,15.2885822331377));
#40796=CARTESIAN_POINT('',(30.,15.0774431706468,15.2885822331377));
#40797=CARTESIAN_POINT('',(30.,15.0774431706468,15.2885822331377));
#40798=CARTESIAN_POINT('Origin',(30.,15.9434685744312,13.7885822331377));
#40799=CARTESIAN_POINT('',(30.,15.9434685744312,13.7885822331377));
#40800=CARTESIAN_POINT('',(30.,15.9434685744312,13.7885822331377));
#40801=CARTESIAN_POINT('',(30.,15.9434685744312,13.7885822331377));
#40802=CARTESIAN_POINT('Origin',(30.,15.0774431706468,12.2885822331377));
#40803=CARTESIAN_POINT('',(30.,15.0774431706468,12.2885822331377));
#40804=CARTESIAN_POINT('',(30.,15.0774431706468,12.2885822331377));
#40805=CARTESIAN_POINT('',(30.,15.0774431706468,12.2885822331377));
#40806=CARTESIAN_POINT('Origin',(30.,13.3453923630779,12.2885822331377));
#40807=CARTESIAN_POINT('',(30.,13.3453923630779,12.2885822331377));
#40808=CARTESIAN_POINT('Origin',(30.,0.,0.));
#40809=CARTESIAN_POINT('Origin',(30.,12.4793669592934,-13.7885822331377));
#40810=CARTESIAN_POINT('',(30.,13.3453923630779,-15.2885822331377));
#40811=CARTESIAN_POINT('',(30.,13.3453923630779,-15.2885822331377));
#40812=CARTESIAN_POINT('',(30.,12.4793669592934,-13.7885822331377));
#40813=CARTESIAN_POINT('',(30.,12.4793669592934,-13.7885822331377));
#40814=CARTESIAN_POINT('',(30.,12.4793669592934,-13.7885822331377));
#40815=CARTESIAN_POINT('Origin',(30.,13.3453923630779,-12.2885822331377));
#40816=CARTESIAN_POINT('',(30.,13.3453923630779,-12.2885822331377));
#40817=CARTESIAN_POINT('',(30.,13.3453923630779,-12.2885822331377));
#40818=CARTESIAN_POINT('',(30.,13.3453923630779,-12.2885822331377));
#40819=CARTESIAN_POINT('Origin',(30.,15.0774431706468,-12.2885822331377));
#40820=CARTESIAN_POINT('',(30.,15.0774431706468,-12.2885822331377));
#40821=CARTESIAN_POINT('',(30.,15.0774431706468,-12.2885822331377));
#40822=CARTESIAN_POINT('',(30.,15.0774431706468,-12.2885822331377));
#40823=CARTESIAN_POINT('Origin',(30.,15.9434685744312,-13.7885822331377));
#40824=CARTESIAN_POINT('',(30.,15.9434685744312,-13.7885822331377));
#40825=CARTESIAN_POINT('',(30.,15.9434685744312,-13.7885822331377));
#40826=CARTESIAN_POINT('',(30.,15.9434685744312,-13.7885822331377));
#40827=CARTESIAN_POINT('Origin',(30.,15.0774431706468,-15.2885822331377));
#40828=CARTESIAN_POINT('',(30.,15.0774431706468,-15.2885822331377));
#40829=CARTESIAN_POINT('',(30.,15.0774431706468,-15.2885822331377));
#40830=CARTESIAN_POINT('',(30.,15.0774431706468,-15.2885822331377));
#40831=CARTESIAN_POINT('Origin',(30.,13.3453923630779,-15.2885822331377));
#40832=CARTESIAN_POINT('',(30.,13.3453923630779,-15.2885822331377));
#40833=CARTESIAN_POINT('Origin',(30.,0.,0.));
#40834=CARTESIAN_POINT('Origin',(2.,42.,0.));
#40835=CARTESIAN_POINT('Origin',(6.,37.75,0.));
#40836=CARTESIAN_POINT('Origin',(24.,35.5,0.));
#40837=CARTESIAN_POINT('Origin',(27.,37.75,0.));
#66660=UNCERTAINTY_MEASURE_WITH_UNIT(LENGTH_MEASURE(0.01),#66722,
'DISTANCE_ACCURACY_VALUE',
'Maximum model space distance between geometric entities at asserted c
onnectivities');
#66680=UNCERTAINTY_MEASURE_WITH_UNIT(LENGTH_MEASURE(0.01),#66722,
'DISTANCE_ACCURACY_VALUE',
'Maximum model space distance between geometric entities at asserted c
onnectivities');
#66701=(
GEOMETRIC_REPRESENTATION_CONTEXT(3)
GLOBAL_UNCERTAINTY_ASSIGNED_CONTEXT((#66660))
GLOBAL_UNIT_ASSIGNED_CONTEXT((#66722,#66724,#66725))
REPRESENTATION_CONTEXT('','3D')
);
#66721=(
GEOMETRIC_REPRESENTATION_CONTEXT(3)
GLOBAL_UNCERTAINTY_ASSIGNED_CONTEXT((#66680))
GLOBAL_UNIT_ASSIGNED_CONTEXT((#66722,#66724,#66725))
REPRESENTATION_CONTEXT('','3D')
);
#66722=(
LENGTH_UNIT()
NAMED_UNIT(*)
SI_UNIT(.MILLI.,.METRE.)
);
#66724=(
NAMED_UNIT(*)
PLANE_ANGLE_UNIT()
SI_UNIT($,.RADIAN.)
);
#66725=(
NAMED_UNIT(*)
SI_UNIT($,.STERADIAN.)
SOLID_ANGLE_UNIT()
);
#66746=SHAPE_DEFINITION_REPRESENTATION(#66802,#66910);
#66802=PRODUCT_DEFINITION_SHAPE('',$,#66951);
#66910=SHAPE_REPRESENTATION('',(#27471),#66701);
#66930=PRODUCT_DEFINITION_CONTEXT('part definition',#67052,'design');
#66951=PRODUCT_DEFINITION('Floating Bearing Housing',
'Floating Bearing Housing',#66991,#66930);
#66991=PRODUCT_DEFINITION_FORMATION('',$,#67074);
#67052=APPLICATION_CONTEXT(
'Core Data for Automotive Mechanical Design Process');
#67053=PRODUCT_CONTEXT('part definition',#67052,'mechanical');
#67074=PRODUCT('Floating Bearing Housing','Floating Bearing Housing',$,
(#67053));
#67095=PRESENTATION_STYLE_ASSIGNMENT((#67097));
#67097=SURFACE_STYLE_USAGE(.BOTH.,#67099);
#67099=SURFACE_SIDE_STYLE('',(#67101));
#67101=SURFACE_STYLE_FILL_AREA(#67103);
#67103=FILL_AREA_STYLE('Opaque(202,209,238)',(#67105));
#67105=FILL_AREA_STYLE_COLOUR('Opaque(202,209,238)',#67107);
#67107=COLOUR_RGB('Opaque(202,209,238)',0.792156862745098,0.819607843137255,
0.933333333333333);
ENDSEC;
END-ISO-10303-21;
